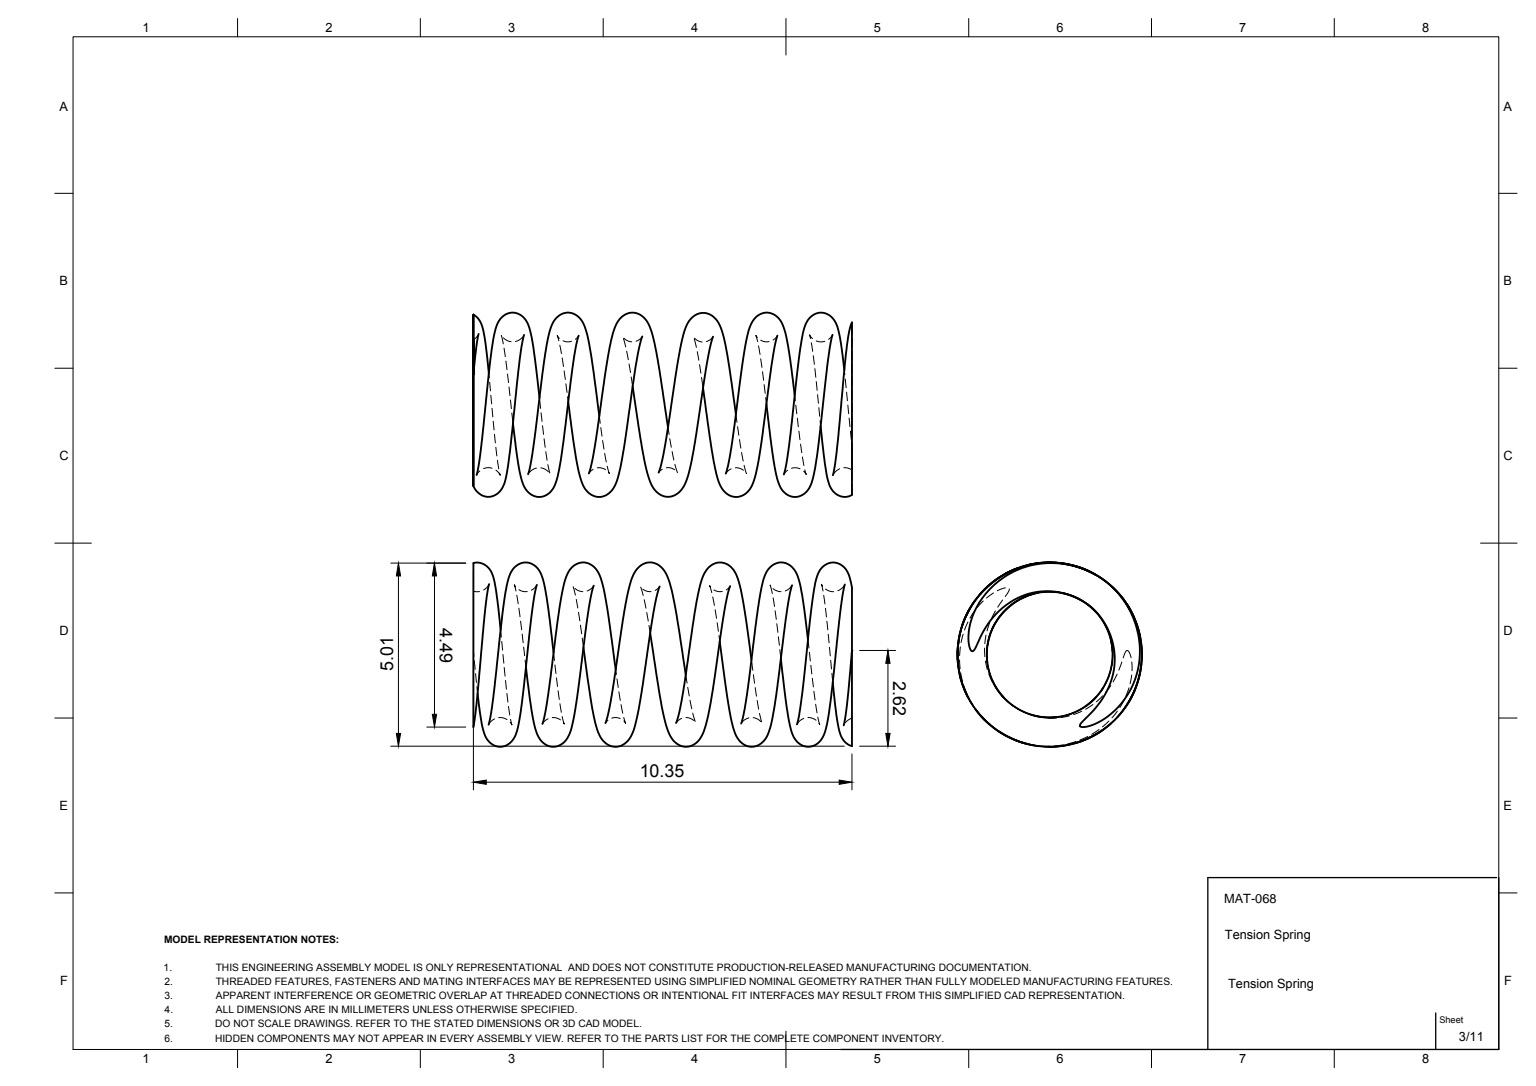
ISO-10303-21;
HEADER;
/* Generated by software containing ST-Developer
 * from STEP Tools, Inc. (www.steptools.com) 
 */

FILE_DESCRIPTION(
/* description */ ('CAx-IF Rec.Pracs.---Representation and Presentation of Product Manufa
cturing Information (PMI)---4.0---2014-10-13'),
/* implementation_level */ '2;1');

FILE_NAME(
/* name */ 'Tension Spring.step',
/* time_stamp */ '2026-10-24T16:53:48-07:00',
/* author */ (''),
/* organization */ (''),
/* preprocessor_version */ 'ST-DEVELOPER v20.2',
/* originating_system */ 'Autodesk Translation Framework v15.17.0.0',
/* authorisation */ '');

FILE_SCHEMA (('AP242_MANAGED_MODEL_BASED_3D_ENGINEERING_MIM_LF { 1 0 10303 442 2 1 4 }'));
ENDSEC;

DATA;
#10=MECHANICAL_DESIGN_GEOMETRIC_PRESENTATION_REPRESENTATION('',(#3490),#107910);
#1137=B_SPLINE_CURVE_WITH_KNOTS('',3,(#63074,#63075,#63076,#63077,#63078,
#63079,#63080,#63081,#63082,#63083,#63084,#63085,#63086,#63087,#63088,#63089,
#63090,#63091,#63092,#63093,#63094,#63095,#63096,#63097,#63098,#63099,#63100,
#63101,#63102,#63103,#63104,#63105,#63106,#63107,#63108,#63109,#63110,#63111,
#63112,#63113,#63114,#63115,#63116,#63117,#63118,#63119,#63120,#63121,#63122,
#63123,#63124,#63125,#63126,#63127,#63128,#63129,#63130,#63131,#63132,#63133,
#63134,#63135,#63136,#63137,#63138,#63139,#63140,#63141,#63142,#63143,#63144,
#63145,#63146,#63147,#63148,#63149,#63150,#63151,#63152,#63153,#63154,#63155,
#63156),.UNSPECIFIED.,.T.,.F.,(4,2,2,2,2,2,2,2,2,2,2,2,3,2,2,2,2,2,2,2,
2,2,2,2,2,2,2,2,2,2,2,2,2,2,2,2,2,2,2,2,4),(-0.599947803193285,-0.598210079042782,
-0.595023554691837,-0.589519553668659,-0.577119648198067,-0.557048780033889,
-0.513453225651634,-0.469622814326577,-0.408953064788174,-0.324588709422408,
-0.21162571525016,-0.096634471246167,0.,0.0616122332173725,0.106433599409592,
0.154580821050161,0.198356973080929,0.2347927451485,0.252280410989761,0.259282926921628,
0.262487356696865,0.264544192713024,0.266469924405381,0.268877657633077,
0.272576047854324,0.281287606126543,0.323717973586198,0.361493711229503,
0.406553787309279,0.452201240933876,0.498262558787684,0.554089254539195,
0.609870344197402,0.658248710788607,0.705297953991042,0.768328967391763,
0.788964957538382,0.796607886518312,0.800333694334371,0.802819259400907,
0.803509190912599),.UNSPECIFIED.);
#1138=B_SPLINE_CURVE_WITH_KNOTS('',3,(#63158,#63159,#63160,#63161,#63162,
#63163,#63164,#63165,#63166,#63167,#63168,#63169,#63170,#63171,#63172,#63173,
#63174,#63175,#63176,#63177,#63178,#63179,#63180,#63181,#63182,#63183,#63184,
#63185,#63186,#63187,#63188,#63189,#63190,#63191,#63192,#63193,#63194,#63195,
#63196,#63197,#63198,#63199,#63200,#63201,#63202,#63203,#63204,#63205,#63206,
#63207,#63208,#63209,#63210,#63211,#63212,#63213,#63214,#63215,#63216,#63217,
#63218,#63219,#63220,#63221,#63222,#63223,#63224,#63225,#63226,#63227,#63228,
#63229,#63230,#63231,#63232,#63233,#63234,#63235,#63236,#63237,#63238,#63239,
#63240,#63241,#63242,#63243,#63244,#63245,#63246,#63247,#63248,#63249,#63250,
#63251,#63252,#63253,#63254,#63255,#63256,#63257,#63258,#63259,#63260,#63261,
#63262,#63263,#63264,#63265,#63266,#63267,#63268,#63269,#63270,#63271,#63272,
#63273),.UNSPECIFIED.,.F.,.F.,(4,2,2,2,2,2,2,2,2,2,2,2,2,2,2,2,2,2,2,2,
2,2,2,2,2,2,2,2,2,2,2,2,2,2,2,2,2,2,2,2,2,2,2,2,2,2,2,2,2,2,2,2,2,2,2,2,
2,4),(-0.961745163027192,-0.959551497797208,-0.949439372246509,-0.939327246695811,
-0.929215121145113,-0.919102995594415,-0.90600602698209,-0.892909058369764,
-0.879812089757439,-0.866715121145113,-0.853618152532788,-0.840521183920462,
-0.827424215308137,-0.814327246695811,-0.801230278083486,-0.78813330947116,
-0.775036340858835,-0.761939372246509,-0.748842403634184,-0.735745435021858,
-0.722648466409533,-0.709551497797208,-0.696454529184882,-0.683357560572557,
-0.670260591960231,-0.657163623347906,-0.630969686123255,-0.604775748898604,
-0.578581811673953,-0.552387874449302,-0.526193937224651,-0.5,-0.484375,
-0.46875,-0.453125,-0.4375,-0.421875,-0.40625,-0.390625,-0.375,-0.359375,
-0.34375,-0.328125,-0.3125,-0.296875,-0.28125,-0.265625,-0.25,-0.234375,
-0.21875,-0.203125,-0.1875,-0.171875,-0.15625,-0.140625,-0.125,-0.109375,
-0.0989179337808057),.UNSPECIFIED.);
#1139=B_SPLINE_CURVE_WITH_KNOTS('',3,(#63275,#63276,#63277,#63278,#63279,
#63280,#63281,#63282,#63283,#63284,#63285,#63286,#63287,#63288,#63289,#63290,
#63291,#63292,#63293,#63294,#63295,#63296,#63297,#63298,#63299,#63300,#63301,
#63302,#63303,#63304,#63305,#63306,#63307,#63308,#63309,#63310,#63311,#63312,
#63313,#63314,#63315,#63316,#63317,#63318,#63319,#63320),.UNSPECIFIED.,
 .F.,.F.,(4,2,2,2,2,2,2,2,2,2,2,2,2,2,2,2,2,2,2,2,2,2,4),(-0.312874562310564,
-0.312343318679824,-0.311777586933697,-0.310438784231193,-0.306394877451961,
-0.293785182499551,-0.270387674138583,-0.246836971206823,-0.225592982310943,
-0.204563523252551,-0.183676969037245,-0.162538995601613,-0.140338814786806,
-0.119352240670363,-0.0971458868601155,-0.0708223711118798,-0.0453771530160624,
-0.0210971413466181,-0.00826159404632588,-0.00338196220690753,-0.00156167910744416,
-0.000763386858963189,-1.00001651581749E-6),.UNSPECIFIED.);
#1140=B_SPLINE_CURVE_WITH_KNOTS('',3,(#63321,#63322,#63323,#63324,#63325,
#63326,#63327,#63328,#63329,#63330,#63331,#63332,#63333,#63334,#63335,#63336,
#63337,#63338,#63339,#63340,#63341,#63342,#63343,#63344,#63345,#63346,#63347,
#63348,#63349,#63350,#63351,#63352,#63353,#63354,#63355,#63356,#63357,#63358,
#63359,#63360,#63361,#63362),.UNSPECIFIED.,.F.,.F.,(4,2,2,2,2,2,2,2,2,2,
2,2,2,2,2,2,2,2,2,2,4),(-0.324422676430501,-0.322867183051822,-0.321207977750209,
-0.317288633341995,-0.30789162270818,-0.28791232922133,-0.250322309326329,
-0.219033304596212,-0.190889649268595,-0.159649528873206,-0.130027804319714,
-0.101827459859418,-0.0752726588112276,-0.0561355587291201,-0.0422771346435577,
-0.0237288423555526,-0.01099220502612,-0.00489383549143937,-0.00219752038096737,
-0.00104712084043852,-1.00002643327324E-6),.UNSPECIFIED.);
#2198=B_SPLINE_SURFACE_WITH_KNOTS('',3,3,((#61813,#61814,#61815,#61816,
#61817,#61818,#61819,#61820,#61821,#61822,#61823,#61824,#61825,#61826,#61827,
#61828,#61829,#61830,#61831,#61832,#61833,#61834,#61835,#61836,#61837,#61838,
#61839,#61840,#61841,#61842,#61843,#61844,#61845,#61846,#61847,#61848,#61849,
#61850,#61851,#61852,#61853,#61854,#61855,#61856,#61857,#61858,#61859,#61860,
#61861,#61862,#61863,#61864,#61865,#61866,#61867,#61868,#61869,#61870,#61871,
#61872,#61873,#61874,#61875,#61876,#61877,#61878,#61879,#61880,#61881,#61882,
#61883,#61884,#61885,#61886,#61887,#61888,#61889,#61890,#61891,#61892,#61893,
#61894,#61895,#61896,#61897,#61898,#61899,#61900,#61901,#61902,#61903,#61904,
#61905,#61906,#61907,#61908,#61909,#61910,#61911,#61912,#61913,#61914,#61915,
#61916,#61917,#61918,#61919,#61920,#61921,#61922,#61923,#61924,#61925,#61926,
#61927,#61928,#61929,#61930,#61931,#61932,#61933,#61934,#61935,#61936,#61937,
#61938),(#61939,#61940,#61941,#61942,#61943,#61944,#61945,#61946,#61947,
#61948,#61949,#61950,#61951,#61952,#61953,#61954,#61955,#61956,#61957,#61958,
#61959,#61960,#61961,#61962,#61963,#61964,#61965,#61966,#61967,#61968,#61969,
#61970,#61971,#61972,#61973,#61974,#61975,#61976,#61977,#61978,#61979,#61980,
#61981,#61982,#61983,#61984,#61985,#61986,#61987,#61988,#61989,#61990,#61991,
#61992,#61993,#61994,#61995,#61996,#61997,#61998,#61999,#62000,#62001,#62002,
#62003,#62004,#62005,#62006,#62007,#62008,#62009,#62010,#62011,#62012,#62013,
#62014,#62015,#62016,#62017,#62018,#62019,#62020,#62021,#62022,#62023,#62024,
#62025,#62026,#62027,#62028,#62029,#62030,#62031,#62032,#62033,#62034,#62035,
#62036,#62037,#62038,#62039,#62040,#62041,#62042,#62043,#62044,#62045,#62046,
#62047,#62048,#62049,#62050,#62051,#62052,#62053,#62054,#62055,#62056,#62057,
#62058,#62059,#62060,#62061,#62062,#62063,#62064),(#62065,#62066,#62067,
#62068,#62069,#62070,#62071,#62072,#62073,#62074,#62075,#62076,#62077,#62078,
#62079,#62080,#62081,#62082,#62083,#62084,#62085,#62086,#62087,#62088,#62089,
#62090,#62091,#62092,#62093,#62094,#62095,#62096,#62097,#62098,#62099,#62100,
#62101,#62102,#62103,#62104,#62105,#62106,#62107,#62108,#62109,#62110,#62111,
#62112,#62113,#62114,#62115,#62116,#62117,#62118,#62119,#62120,#62121,#62122,
#62123,#62124,#62125,#62126,#62127,#62128,#62129,#62130,#62131,#62132,#62133,
#62134,#62135,#62136,#62137,#62138,#62139,#62140,#62141,#62142,#62143,#62144,
#62145,#62146,#62147,#62148,#62149,#62150,#62151,#62152,#62153,#62154,#62155,
#62156,#62157,#62158,#62159,#62160,#62161,#62162,#62163,#62164,#62165,#62166,
#62167,#62168,#62169,#62170,#62171,#62172,#62173,#62174,#62175,#62176,#62177,
#62178,#62179,#62180,#62181,#62182,#62183,#62184,#62185,#62186,#62187,#62188,
#62189,#62190),(#62191,#62192,#62193,#62194,#62195,#62196,#62197,#62198,
#62199,#62200,#62201,#62202,#62203,#62204,#62205,#62206,#62207,#62208,#62209,
#62210,#62211,#62212,#62213,#62214,#62215,#62216,#62217,#62218,#62219,#62220,
#62221,#62222,#62223,#62224,#62225,#62226,#62227,#62228,#62229,#62230,#62231,
#62232,#62233,#62234,#62235,#62236,#62237,#62238,#62239,#62240,#62241,#62242,
#62243,#62244,#62245,#62246,#62247,#62248,#62249,#62250,#62251,#62252,#62253,
#62254,#62255,#62256,#62257,#62258,#62259,#62260,#62261,#62262,#62263,#62264,
#62265,#62266,#62267,#62268,#62269,#62270,#62271,#62272,#62273,#62274,#62275,
#62276,#62277,#62278,#62279,#62280,#62281,#62282,#62283,#62284,#62285,#62286,
#62287,#62288,#62289,#62290,#62291,#62292,#62293,#62294,#62295,#62296,#62297,
#62298,#62299,#62300,#62301,#62302,#62303,#62304,#62305,#62306,#62307,#62308,
#62309,#62310,#62311,#62312,#62313,#62314,#62315,#62316),(#62317,#62318,
#62319,#62320,#62321,#62322,#62323,#62324,#62325,#62326,#62327,#62328,#62329,
#62330,#62331,#62332,#62333,#62334,#62335,#62336,#62337,#62338,#62339,#62340,
#62341,#62342,#62343,#62344,#62345,#62346,#62347,#62348,#62349,#62350,#62351,
#62352,#62353,#62354,#62355,#62356,#62357,#62358,#62359,#62360,#62361,#62362,
#62363,#62364,#62365,#62366,#62367,#62368,#62369,#62370,#62371,#62372,#62373,
#62374,#62375,#62376,#62377,#62378,#62379,#62380,#62381,#62382,#62383,#62384,
#62385,#62386,#62387,#62388,#62389,#62390,#62391,#62392,#62393,#62394,#62395,
#62396,#62397,#62398,#62399,#62400,#62401,#62402,#62403,#62404,#62405,#62406,
#62407,#62408,#62409,#62410,#62411,#62412,#62413,#62414,#62415,#62416,#62417,
#62418,#62419,#62420,#62421,#62422,#62423,#62424,#62425,#62426,#62427,#62428,
#62429,#62430,#62431,#62432,#62433,#62434,#62435,#62436,#62437,#62438,#62439,
#62440,#62441,#62442),(#62443,#62444,#62445,#62446,#62447,#62448,#62449,
#62450,#62451,#62452,#62453,#62454,#62455,#62456,#62457,#62458,#62459,#62460,
#62461,#62462,#62463,#62464,#62465,#62466,#62467,#62468,#62469,#62470,#62471,
#62472,#62473,#62474,#62475,#62476,#62477,#62478,#62479,#62480,#62481,#62482,
#62483,#62484,#62485,#62486,#62487,#62488,#62489,#62490,#62491,#62492,#62493,
#62494,#62495,#62496,#62497,#62498,#62499,#62500,#62501,#62502,#62503,#62504,
#62505,#62506,#62507,#62508,#62509,#62510,#62511,#62512,#62513,#62514,#62515,
#62516,#62517,#62518,#62519,#62520,#62521,#62522,#62523,#62524,#62525,#62526,
#62527,#62528,#62529,#62530,#62531,#62532,#62533,#62534,#62535,#62536,#62537,
#62538,#62539,#62540,#62541,#62542,#62543,#62544,#62545,#62546,#62547,#62548,
#62549,#62550,#62551,#62552,#62553,#62554,#62555,#62556,#62557,#62558,#62559,
#62560,#62561,#62562,#62563,#62564,#62565,#62566,#62567,#62568),(#62569,
#62570,#62571,#62572,#62573,#62574,#62575,#62576,#62577,#62578,#62579,#62580,
#62581,#62582,#62583,#62584,#62585,#62586,#62587,#62588,#62589,#62590,#62591,
#62592,#62593,#62594,#62595,#62596,#62597,#62598,#62599,#62600,#62601,#62602,
#62603,#62604,#62605,#62606,#62607,#62608,#62609,#62610,#62611,#62612,#62613,
#62614,#62615,#62616,#62617,#62618,#62619,#62620,#62621,#62622,#62623,#62624,
#62625,#62626,#62627,#62628,#62629,#62630,#62631,#62632,#62633,#62634,#62635,
#62636,#62637,#62638,#62639,#62640,#62641,#62642,#62643,#62644,#62645,#62646,
#62647,#62648,#62649,#62650,#62651,#62652,#62653,#62654,#62655,#62656,#62657,
#62658,#62659,#62660,#62661,#62662,#62663,#62664,#62665,#62666,#62667,#62668,
#62669,#62670,#62671,#62672,#62673,#62674,#62675,#62676,#62677,#62678,#62679,
#62680,#62681,#62682,#62683,#62684,#62685,#62686,#62687,#62688,#62689,#62690,
#62691,#62692,#62693,#62694),(#62695,#62696,#62697,#62698,#62699,#62700,
#62701,#62702,#62703,#62704,#62705,#62706,#62707,#62708,#62709,#62710,#62711,
#62712,#62713,#62714,#62715,#62716,#62717,#62718,#62719,#62720,#62721,#62722,
#62723,#62724,#62725,#62726,#62727,#62728,#62729,#62730,#62731,#62732,#62733,
#62734,#62735,#62736,#62737,#62738,#62739,#62740,#62741,#62742,#62743,#62744,
#62745,#62746,#62747,#62748,#62749,#62750,#62751,#62752,#62753,#62754,#62755,
#62756,#62757,#62758,#62759,#62760,#62761,#62762,#62763,#62764,#62765,#62766,
#62767,#62768,#62769,#62770,#62771,#62772,#62773,#62774,#62775,#62776,#62777,
#62778,#62779,#62780,#62781,#62782,#62783,#62784,#62785,#62786,#62787,#62788,
#62789,#62790,#62791,#62792,#62793,#62794,#62795,#62796,#62797,#62798,#62799,
#62800,#62801,#62802,#62803,#62804,#62805,#62806,#62807,#62808,#62809,#62810,
#62811,#62812,#62813,#62814,#62815,#62816,#62817,#62818,#62819,#62820),
(#62821,#62822,#62823,#62824,#62825,#62826,#62827,#62828,#62829,#62830,
#62831,#62832,#62833,#62834,#62835,#62836,#62837,#62838,#62839,#62840,#62841,
#62842,#62843,#62844,#62845,#62846,#62847,#62848,#62849,#62850,#62851,#62852,
#62853,#62854,#62855,#62856,#62857,#62858,#62859,#62860,#62861,#62862,#62863,
#62864,#62865,#62866,#62867,#62868,#62869,#62870,#62871,#62872,#62873,#62874,
#62875,#62876,#62877,#62878,#62879,#62880,#62881,#62882,#62883,#62884,#62885,
#62886,#62887,#62888,#62889,#62890,#62891,#62892,#62893,#62894,#62895,#62896,
#62897,#62898,#62899,#62900,#62901,#62902,#62903,#62904,#62905,#62906,#62907,
#62908,#62909,#62910,#62911,#62912,#62913,#62914,#62915,#62916,#62917,#62918,
#62919,#62920,#62921,#62922,#62923,#62924,#62925,#62926,#62927,#62928,#62929,
#62930,#62931,#62932,#62933,#62934,#62935,#62936,#62937,#62938,#62939,#62940,
#62941,#62942,#62943,#62944,#62945,#62946),(#62947,#62948,#62949,#62950,
#62951,#62952,#62953,#62954,#62955,#62956,#62957,#62958,#62959,#62960,#62961,
#62962,#62963,#62964,#62965,#62966,#62967,#62968,#62969,#62970,#62971,#62972,
#62973,#62974,#62975,#62976,#62977,#62978,#62979,#62980,#62981,#62982,#62983,
#62984,#62985,#62986,#62987,#62988,#62989,#62990,#62991,#62992,#62993,#62994,
#62995,#62996,#62997,#62998,#62999,#63000,#63001,#63002,#63003,#63004,#63005,
#63006,#63007,#63008,#63009,#63010,#63011,#63012,#63013,#63014,#63015,#63016,
#63017,#63018,#63019,#63020,#63021,#63022,#63023,#63024,#63025,#63026,#63027,
#63028,#63029,#63030,#63031,#63032,#63033,#63034,#63035,#63036,#63037,#63038,
#63039,#63040,#63041,#63042,#63043,#63044,#63045,#63046,#63047,#63048,#63049,
#63050,#63051,#63052,#63053,#63054,#63055,#63056,#63057,#63058,#63059,#63060,
#63061,#63062,#63063,#63064,#63065,#63066,#63067,#63068,#63069,#63070,#63071,
#63072)),.UNSPECIFIED.,.T.,.F.,.F.,(4,2,2,2,4),(4,2,2,2,2,2,2,2,2,2,2,2,
2,2,2,2,2,2,2,2,2,2,2,2,2,2,2,2,2,2,2,2,2,2,2,2,2,2,2,2,2,2,2,2,2,2,2,2,
2,2,2,2,2,2,2,2,2,2,2,2,2,2,4),(0.,0.25,0.5,0.75,1.),(0.0266743037386738,
0.03125,0.046875,0.0625,0.078125,0.09375,0.109375,0.125,0.140625,0.15625,
0.171875,0.1875,0.203125,0.21875,0.234375,0.25,0.265625,0.28125,0.296875,
0.3125,0.328125,0.34375,0.359375,0.375,0.390625,0.40625,0.421875,0.4375,
0.453125,0.46875,0.484375,0.5,0.526193937224651,0.552387874449302,0.578581811673953,
0.604775748898604,0.630969686123255,0.657163623347906,0.670260591960231,
0.683357560572557,0.696454529184882,0.709551497797208,0.722648466409533,
0.735745435021858,0.748842403634184,0.761939372246509,0.775036340858835,
0.78813330947116,0.801230278083486,0.814327246695811,0.827424215308137,
0.840521183920462,0.853618152532788,0.866715121145113,0.879812089757439,
0.892909058369764,0.90600602698209,0.919102995594415,0.929215121145113,
0.939327246695811,0.949439372246509,0.959551497797208,0.967322126402602),
 .UNSPECIFIED.);
#3470=SHAPE_REPRESENTATION_RELATIONSHIP('SRR','None',#107948,#3480);
#3480=ADVANCED_BREP_SHAPE_REPRESENTATION('',(#3500),#107901);
#3490=STYLED_ITEM('',(#108007),#3500);
#3500=MANIFOLD_SOLID_BREP('Body1',#45538);
#3544=PLANE('',#45669);
#3545=PLANE('',#45670);
#3762=FACE_OUTER_BOUND('',#6688,.T.);
#3763=FACE_OUTER_BOUND('',#6689,.T.);
#3764=FACE_OUTER_BOUND('',#6690,.T.);
#6688=EDGE_LOOP('',(#28134,#28135,#28136,#28137,#28138));
#6689=EDGE_LOOP('',(#28139,#28140));
#6690=EDGE_LOOP('',(#28141));
#17183=VERTEX_POINT('',#63073);
#17184=VERTEX_POINT('',#63157);
#17185=VERTEX_POINT('',#63274);
#21209=EDGE_CURVE('',#17183,#17183,#1137,.F.);
#21210=EDGE_CURVE('',#17183,#17184,#1138,.T.);
#21211=EDGE_CURVE('',#17184,#17185,#1139,.F.);
#21212=EDGE_CURVE('',#17185,#17184,#1140,.F.);
#28134=ORIENTED_EDGE('',*,*,#21209,.T.);
#28135=ORIENTED_EDGE('',*,*,#21210,.T.);
#28136=ORIENTED_EDGE('',*,*,#21211,.T.);
#28137=ORIENTED_EDGE('',*,*,#21212,.T.);
#28138=ORIENTED_EDGE('',*,*,#21210,.F.);
#28139=ORIENTED_EDGE('',*,*,#21211,.F.);
#28140=ORIENTED_EDGE('',*,*,#21212,.F.);
#28141=ORIENTED_EDGE('',*,*,#21209,.F.);
#42617=ADVANCED_FACE('',(#3762),#2198,.T.);
#42618=ADVANCED_FACE('',(#3763),#3544,.T.);
#42619=ADVANCED_FACE('',(#3764),#3545,.T.);
#45538=CLOSED_SHELL('',(#42617,#42618,#42619));
#45668=AXIS2_PLACEMENT_3D('',#61812,#50398,#50399);
#45669=AXIS2_PLACEMENT_3D('',#63363,#50400,#50401);
#45670=AXIS2_PLACEMENT_3D('',#63364,#50402,#50403);
#50398=DIRECTION('axis',(0.,0.,1.));
#50399=DIRECTION('refdir',(1.,0.,0.));
#50400=DIRECTION('center_axis',(-3.37541892033393E-34,1.,-4.11561597259898E-17));
#50401=DIRECTION('ref_axis',(1.,-1.28292706084425E-49,-8.20149144819841E-18));
#50402=DIRECTION('center_axis',(-1.19904736293711E-16,-1.,2.51898569257898E-21));
#50403=DIRECTION('ref_axis',(-1.,1.19904736293711E-16,0.));
#61812=CARTESIAN_POINT('',(0.,0.,0.));
#61813=CARTESIAN_POINT('Ctrl Pts',(0.00815067148752137,-0.0203072579114564,
0.0762656663521488));
#61814=CARTESIAN_POINT('Ctrl Pts',(0.0083771381325318,-0.0203255606965017,
0.0762649347079084));
#61815=CARTESIAN_POINT('Ctrl Pts',(0.00860198035030984,-0.0203438634815471,
0.0762288078613937));
#61816=CARTESIAN_POINT('Ctrl Pts',(0.00953656982276594,-0.0204246662665928,
0.0759073888491967));
#61817=CARTESIAN_POINT('Ctrl Pts',(0.0100801851138304,-0.0204871662665918,
0.0752518676024789));
#61818=CARTESIAN_POINT('Ctrl Pts',(0.0103422385382883,-0.0206121662665931,
0.0738034800723812));
#61819=CARTESIAN_POINT('Ctrl Pts',(0.0100648920002843,-0.020674666266593,
0.0730378901277388));
#61820=CARTESIAN_POINT('Ctrl Pts',(0.00900362893656076,-0.0207996662665919,
0.0720931661776728));
#61821=CARTESIAN_POINT('Ctrl Pts',(0.008241028020177,-0.0208621662665925,
0.0719231783970233));
#61822=CARTESIAN_POINT('Ctrl Pts',(0.00691275415584957,-0.0209871662665924,
0.0722775972279668));
#61823=CARTESIAN_POINT('Ctrl Pts',(0.00636364311727103,-0.0210496662665924,
0.0727913084945308));
#61824=CARTESIAN_POINT('Ctrl Pts',(0.00590286642913209,-0.0211746662665925,
0.0740419937307385));
#61825=CARTESIAN_POINT('Ctrl Pts',(0.00599202908596152,-0.0212371662665924,
0.0747620631556615));
#61826=CARTESIAN_POINT('Ctrl Pts',(0.00669689975963152,-0.0213621662665925,
0.0758479396774564));
#61827=CARTESIAN_POINT('Ctrl Pts',(0.00730138706368173,-0.0214246662665922,
0.0762043156608544));
#61828=CARTESIAN_POINT('Ctrl Pts',(0.00855547426588603,-0.0215496662665927,
0.0763202968801402));
#61829=CARTESIAN_POINT('Ctrl Pts',(0.00919252612250013,-0.0216121662665926,
0.0760823999614819));
#61830=CARTESIAN_POINT('Ctrl Pts',(0.0100589999732895,-0.0217371662665924,
0.075213633090309));
#61831=CARTESIAN_POINT('Ctrl Pts',(0.0102830084237745,-0.0217996662665926,
0.0745926208223076));
#61832=CARTESIAN_POINT('Ctrl Pts',(0.0101959629269755,-0.0219246662665924,
0.0733988421450626));
#61833=CARTESIAN_POINT('Ctrl Pts',(0.00988830420246689,-0.0219871662665922,
0.0728354269849725));
#61834=CARTESIAN_POINT('Ctrl Pts',(0.00896597799697031,-0.0221121662665928,
0.0721171826520367));
#61835=CARTESIAN_POINT('Ctrl Pts',(0.00835948988205837,-0.022174666266592,
0.0719657358996911));
#61836=CARTESIAN_POINT('Ctrl Pts',(0.00723038395375605,-0.0222996662665929,
0.0721429107222321));
#61837=CARTESIAN_POINT('Ctrl Pts',(0.00671499560243656,-0.0223621662665927,
0.0724683075554325));
#61838=CARTESIAN_POINT('Ctrl Pts',(0.00606901592181546,-0.0224871662665922,
0.0733814268319492));
#61839=CARTESIAN_POINT('Ctrl Pts',(0.00594091088577522,-0.0225496662665926,
0.0739624842354635));
#61840=CARTESIAN_POINT('Ctrl Pts',(0.00612305344798784,-0.0226746662665923,
0.0750428459007938));
#61841=CARTESIAN_POINT('Ctrl Pts',(0.00643067872875265,-0.0227371662665921,
0.0755362893544149));
#61842=CARTESIAN_POINT('Ctrl Pts',(0.00729424742007936,-0.0228621662665928,
0.0761749122408133));
#61843=CARTESIAN_POINT('Ctrl Pts',(0.00784480408877878,-0.0229246662665925,
0.0763178915621161));
#61844=CARTESIAN_POINT('Ctrl Pts',(0.00889151097164585,-0.0230496662665924,
0.0761965031486893));
#61845=CARTESIAN_POINT('Ctrl Pts',(0.00938270763587042,-0.0231121662665924,
0.0759340000649118));
#61846=CARTESIAN_POINT('Ctrl Pts',(0.0100625879641978,-0.0232371662665925,
0.0751542816790953));
#61847=CARTESIAN_POINT('Ctrl Pts',(0.0102490546008787,-0.0232996662665926,
0.0746413589041057));
#61848=CARTESIAN_POINT('Ctrl Pts',(0.0102410178141923,-0.0234246662665924,
0.0736250907589115));
#61849=CARTESIAN_POINT('Ctrl Pts',(0.0100475843126518,-0.0234871662665927,
0.0731260381541277));
#61850=CARTESIAN_POINT('Ctrl Pts',(0.00938855725198137,-0.0236121662665922,
0.0723752164881653));
#61851=CARTESIAN_POINT('Ctrl Pts',(0.0089262758271642,-0.0236746662665927,
0.0721258013564626));
#61852=CARTESIAN_POINT('Ctrl Pts',(0.00795468689116961,-0.0237996662665922,
0.0719791054916663));
#61853=CARTESIAN_POINT('Ctrl Pts',(0.00744911026789867,-0.0238621662665923,
0.0720815291713897));
#61854=CARTESIAN_POINT('Ctrl Pts',(0.00661942895548025,-0.0239871662665926,
0.0725781618664859));
#61855=CARTESIAN_POINT('Ctrl Pts',(0.00629781787585632,-0.0240496662665925,
0.0729699778138594));
#61856=CARTESIAN_POINT('Ctrl Pts',(0.00596869167054677,-0.0241746662665925,
0.07386332441141));
#61857=CARTESIAN_POINT('Ctrl Pts',(0.00596159400885685,-0.0242371662665925,
0.0743616829432692));
#61858=CARTESIAN_POINT('Ctrl Pts',(0.00625226027464946,-0.0243621662665925,
0.0752533010137793));
#61859=CARTESIAN_POINT('Ctrl Pts',(0.0065485129249735,-0.0244246662665925,
0.0756440052932471));
#61860=CARTESIAN_POINT('Ctrl Pts',(0.00731262787164867,-0.0245496662665925,
0.0761638405487234));
#61861=CARTESIAN_POINT('Ctrl Pts',(0.00777792798085125,-0.0246121662665926,
0.0762919438047406));
#61862=CARTESIAN_POINT('Ctrl Pts',(0.00868784969457759,-0.0247371662665924,
0.07624508144423));
#61863=CARTESIAN_POINT('Ctrl Pts',(0.00912998835433636,-0.024799666266592,
0.0760707882292855));
#61864=CARTESIAN_POINT('Ctrl Pts',(0.00982231809848441,-0.024924666266593,
0.07549790728317));
#61865=CARTESIAN_POINT('Ctrl Pts',(0.010071019077723,-0.0249871662665926,
0.0751012030151419));
#61866=CARTESIAN_POINT('Ctrl Pts',(0.0102889821151069,-0.0251121662665924,
0.0742418039415068));
#61867=CARTESIAN_POINT('Ctrl Pts',(0.0102581523851926,-0.0251746662665924,
0.0737813536046464));
#61868=CARTESIAN_POINT('Ctrl Pts',(0.00993809892066803,-0.0252996662665926,
0.0729669145852015));
#61869=CARTESIAN_POINT('Ctrl Pts',(0.00965002750714532,-0.0253621662665928,
0.0726146871985494));
#61870=CARTESIAN_POINT('Ctrl Pts',(0.00892808254078336,-0.0254871662665921,
0.07214009674052));
#61871=CARTESIAN_POINT('Ctrl Pts',(0.00849604407482765,-0.0255496662665926,
0.0720184647612599));
#61872=CARTESIAN_POINT('Ctrl Pts',(0.00764304374228332,-0.0256746662665924,
0.0720402815521564));
#61873=CARTESIAN_POINT('Ctrl Pts',(0.00722389165927775,-0.0257371662665915,
0.0721833149981475));
#61874=CARTESIAN_POINT('Ctrl Pts',(0.00654039915241529,-0.0258621662665935,
0.0726767209970879));
#61875=CARTESIAN_POINT('Ctrl Pts',(0.00627724799864211,-0.0259246662665926,
0.0730258105884879));
#61876=CARTESIAN_POINT('Ctrl Pts',(0.00589186280469173,-0.0260919420154909,
0.0740718608505132));
#61877=CARTESIAN_POINT('Ctrl Pts',(0.00599991759097347,-0.0261967177643892,
0.0748547737082654));
#61878=CARTESIAN_POINT('Ctrl Pts',(0.00685580966361203,-0.0264062692621874,
0.0759938417732247));
#61879=CARTESIAN_POINT('Ctrl Pts',(0.00759343482402584,-0.0265110450110865,
0.0763289629385248));
#61880=CARTESIAN_POINT('Ctrl Pts',(0.00904218730885863,-0.0267205965088817,
0.0761958934123178));
#61881=CARTESIAN_POINT('Ctrl Pts',(0.00972755157183108,-0.0268253722577806,
0.0757250048942655));
#61882=CARTESIAN_POINT('Ctrl Pts',(0.010359884849577,-0.0270349237555792,
0.0743792630330001));
#61883=CARTESIAN_POINT('Ctrl Pts',(0.0102896623256786,-0.0271396995044774,
0.0735275482799331));
#61884=CARTESIAN_POINT('Ctrl Pts',(0.00940073146439328,-0.0273492510022741,
0.0722931522835415));
#61885=CARTESIAN_POINT('Ctrl Pts',(0.00859517611493118,-0.0274540267511745,
0.0719398966766563));
#61886=CARTESIAN_POINT('Ctrl Pts',(0.00705289958900958,-0.0276635782489686,
0.0721600303097132));
#61887=CARTESIAN_POINT('Ctrl Pts',(0.00635232687879448,-0.0277683539978693,
0.0727358184526565));
#61888=CARTESIAN_POINT('Ctrl Pts',(0.00598272505460037,-0.0279255176212164,
0.073875472823177));
#61889=CARTESIAN_POINT('Ctrl Pts',(0.00596897958949985,-0.0279779054956661,
0.0742932638294421));
#61890=CARTESIAN_POINT('Ctrl Pts',(0.00617298034709087,-0.0280826812445643,
0.0750763211850444));
#61891=CARTESIAN_POINT('Ctrl Pts',(0.00639068647810172,-0.0281350691190143,
0.075440160464901));
#61892=CARTESIAN_POINT('Ctrl Pts',(0.00699633121784709,-0.028239844867912,
0.0759930922591544));
#61893=CARTESIAN_POINT('Ctrl Pts',(0.00738340683150901,-0.0282922327423619,
0.0761809264433306));
#61894=CARTESIAN_POINT('Ctrl Pts',(0.00820473003409823,-0.0283970084912602,
0.076310154007468));
#61895=CARTESIAN_POINT('Ctrl Pts',(0.00863746583537968,-0.0284493963657099,
0.0762509280036797));
#61896=CARTESIAN_POINT('Ctrl Pts',(0.00940183247449225,-0.0285541721146081,
0.0758948085378461));
#61897=CARTESIAN_POINT('Ctrl Pts',(0.00973174559026465,-0.028606559989058,
0.0755982633195131));
#61898=CARTESIAN_POINT('Ctrl Pts',(0.0101673721494254,-0.0287113357379557,
0.0748618658679991));
#61899=CARTESIAN_POINT('Ctrl Pts',(0.0102717693088642,-0.0287637236124047,
0.0744233616342778));
#61900=CARTESIAN_POINT('Ctrl Pts',(0.0102064021029961,-0.0288684993613048,
0.0735573200377487));
#61901=CARTESIAN_POINT('Ctrl Pts',(0.0100362994783456,-0.0289208872357529,
0.0731317839731108));
#61902=CARTESIAN_POINT('Ctrl Pts',(0.00947201428442268,-0.0290256629846524,
0.072453899629834));
#61903=CARTESIAN_POINT('Ctrl Pts',(0.00907878062310723,-0.0290780508591023,
0.0722035268267701));
#61904=CARTESIAN_POINT('Ctrl Pts',(0.00821001945932422,-0.0291828266079989,
0.0719835875408627));
#61905=CARTESIAN_POINT('Ctrl Pts',(0.00773657577545569,-0.0292352144824501,
0.0720151544508798));
#61906=CARTESIAN_POINT('Ctrl Pts',(0.00689428236856863,-0.0293399902313469,
0.0723623130857159));
#61907=CARTESIAN_POINT('Ctrl Pts',(0.00652798278812114,-0.029392378105796,
0.0726775538261953));
#61908=CARTESIAN_POINT('Ctrl Pts',(0.00605938394721744,-0.0294971538546968,
0.0734769967671513));
#61909=CARTESIAN_POINT('Ctrl Pts',(0.00595907161542407,-0.0295495417291453,
0.0739592244029917));
#61910=CARTESIAN_POINT('Ctrl Pts',(0.00608211280228693,-0.0296543174780434,
0.0748942803942386));
#61911=CARTESIAN_POINT('Ctrl Pts',(0.00630586837465766,-0.0297067053524937,
0.0753440780020337));
#61912=CARTESIAN_POINT('Ctrl Pts',(0.00699741885923872,-0.0298114811013907,
0.0760106285387534));
#61913=CARTESIAN_POINT('Ctrl Pts',(0.00746350290246076,-0.02986386897584,
0.0762245043065757));
#61914=CARTESIAN_POINT('Ctrl Pts',(0.00843911221849071,-0.0299686447247403,
0.0763040900230327));
#61915=CARTESIAN_POINT('Ctrl Pts',(0.0089451874363639,-0.0300210325991884,
0.0761685265237053));
#61916=CARTESIAN_POINT('Ctrl Pts',(0.00975909850238958,-0.0301258083480876,
0.0755904500898765));
#61917=CARTESIAN_POINT('Ctrl Pts',(0.0100631115942824,-0.0301781962225362,
0.0751492903863319));
#61918=CARTESIAN_POINT('Ctrl Pts',(0.0103054074683059,-0.0302829719714357,
0.0741595369305542));
#61919=CARTESIAN_POINT('Ctrl Pts',(0.0102414483775728,-0.0303353598458849,
0.0736148328055268));
#61920=CARTESIAN_POINT('Ctrl Pts',(0.00975323921825422,-0.0304401355947827,
0.0726954265952984));
#61921=CARTESIAN_POINT('Ctrl Pts',(0.00932997882757754,-0.0304925234692313,
0.0723256171343211));
#61922=CARTESIAN_POINT('Ctrl Pts',(0.00832584380498464,-0.0305972992181321,
0.0719722823282605));
#61923=CARTESIAN_POINT('Ctrl Pts',(0.0077494649754808,-0.0306496870925817,
0.0719920559628832));
#61924=CARTESIAN_POINT('Ctrl Pts',(0.00675592000443203,-0.0307544628414776,
0.0724395062495526));
#61925=CARTESIAN_POINT('Ctrl Pts',(0.00634496891942769,-0.0308068507159279,
0.0728664214919276));
#61926=CARTESIAN_POINT('Ctrl Pts',(0.00594354974162806,-0.0309116264648272,
0.0739084696771727));
#61927=CARTESIAN_POINT('Ctrl Pts',(0.00595750536674637,-0.030964014339277,
0.0745180867156372));
#61928=CARTESIAN_POINT('Ctrl Pts',(0.00638267793035737,-0.0310568507159276,
0.0754400513829074));
#61929=CARTESIAN_POINT('Ctrl Pts',(0.00669956413626623,-0.0310972992181319,
0.0757857300068678));
#61930=CARTESIAN_POINT('Ctrl Pts',(0.00748945302262128,-0.0311781962225358,
0.0762240386264647));
#61931=CARTESIAN_POINT('Ctrl Pts',(0.00796079155782699,-0.0312186447247393,
0.0763148367595518));
#61932=CARTESIAN_POINT('Ctrl Pts',(0.00887509295304323,-0.0312995417291452,
0.0761868152287656));
#61933=CARTESIAN_POINT('Ctrl Pts',(0.00931534986442847,-0.031339990231348,
0.075967462485304));
#61934=CARTESIAN_POINT('Ctrl Pts',(0.00997379973563606,-0.0314208872357532,
0.0752903676969252));
#61935=CARTESIAN_POINT('Ctrl Pts',(0.0101892230058022,-0.0314613357379553,
0.0748339923228011));
#61936=CARTESIAN_POINT('Ctrl Pts',(0.0102708978512695,-0.0315328667545812,
0.0739826395793677));
#61937=CARTESIAN_POINT('Ctrl Pts',(0.0102055680523813,-0.0315639492690025,
0.0735997686615574));
#61938=CARTESIAN_POINT('Ctrl Pts',(0.0100469390803206,-0.0315950317834238,
0.0732561803273014));
#61939=CARTESIAN_POINT('Ctrl Pts',(0.00815332628724061,-0.0203072579114564,
0.0764745476396777));
#61940=CARTESIAN_POINT('Ctrl Pts',(0.00840215214987724,-0.0203255606965017,
0.0764737437596658));
#61941=CARTESIAN_POINT('Ctrl Pts',(0.00864919320439181,-0.0203438634815471,
0.0764340500831514));
#61942=CARTESIAN_POINT('Ctrl Pts',(0.00967605537954476,-0.0204246662665928,
0.0760808971366146));
#61943=CARTESIAN_POINT('Ctrl Pts',(0.0102733422062002,-0.0204871662665918,
0.0753606557973937));
#61944=CARTESIAN_POINT('Ctrl Pts',(0.0105612683570671,-0.0206121662665931,
0.0737692679062889));
#61945=CARTESIAN_POINT('Ctrl Pts',(0.0102565391923597,-0.020674666266593,
0.0729280907060315));
#61946=CARTESIAN_POINT('Ctrl Pts',(0.00909049684955361,-0.0207996662665919,
0.0718900934688763));
#61947=CARTESIAN_POINT('Ctrl Pts',(0.00825260378650262,-0.0208621662665925,
0.0717033226702191));
#61948=CARTESIAN_POINT('Ctrl Pts',(0.00679318847130807,-0.0209871662665924,
0.0720927335317618));
#61949=CARTESIAN_POINT('Ctrl Pts',(0.00618986329796383,-0.0210496662665924,
0.0726571638876892));
#61950=CARTESIAN_POINT('Ctrl Pts',(0.00568359379013531,-0.0211746662665925,
0.0740313301927182));
#61951=CARTESIAN_POINT('Ctrl Pts',(0.00578155954133694,-0.0212371662665924,
0.0748224925990252));
#61952=CARTESIAN_POINT('Ctrl Pts',(0.00655602261255478,-0.0213621662665925,
0.076015578504634));
#61953=CARTESIAN_POINT('Ctrl Pts',(0.00722019139059382,-0.0214246662665922,
0.0764071397497255));
#61954=CARTESIAN_POINT('Ctrl Pts',(0.00859809554021233,-0.0215496662665927,
0.0765345718796849));
#61955=CARTESIAN_POINT('Ctrl Pts',(0.00929804399292574,-0.0216121662665926,
0.0762731872241167));
#61956=CARTESIAN_POINT('Ctrl Pts',(0.010250065441227,-0.0217371662665924,
0.0753186463638511));
#61957=CARTESIAN_POINT('Ctrl Pts',(0.0104961904099933,-0.0217996662665926,
0.0746363211000744));
#61958=CARTESIAN_POINT('Ctrl Pts',(0.0104005508475817,-0.0219246662665924,
0.0733246797802278));
#61959=CARTESIAN_POINT('Ctrl Pts',(0.0100625167520088,-0.0219871662665922,
0.0727056382289851));
#61960=CARTESIAN_POINT('Ctrl Pts',(0.00904912860513842,-0.0221121662665928,
0.0719164811073332));
#61961=CARTESIAN_POINT('Ctrl Pts',(0.00838276147471677,-0.022174666266592,
0.0717500819062757));
#61962=CARTESIAN_POINT('Ctrl Pts',(0.00714217809165384,-0.0222996662665929,
0.0719447493287309));
#61963=CARTESIAN_POINT('Ctrl Pts',(0.0065759050711654,-0.0223621662665927,
0.0723022728294504));
#61964=CARTESIAN_POINT('Ctrl Pts',(0.00586614734384593,-0.0224871662665922,
0.0733055450405034));
#61965=CARTESIAN_POINT('Ctrl Pts',(0.00572539440382979,-0.0225496662665926,
0.073943970666777));
#61966=CARTESIAN_POINT('Ctrl Pts',(0.00592552003453053,-0.0226746662665923,
0.0751309972301058));
#61967=CARTESIAN_POINT('Ctrl Pts',(0.00626351738443437,-0.0227371662665921,
0.0756731587170833));
#61968=CARTESIAN_POINT('Ctrl Pts',(0.00721234684475271,-0.0228621662665928,
0.0763748333085017));
#61969=CARTESIAN_POINT('Ctrl Pts',(0.00781726037633776,-0.0229246662665925,
0.0765319290828517));
#61970=CARTESIAN_POINT('Ctrl Pts',(0.00896730939589689,-0.0230496662665924,
0.076398555902516));
#61971=CARTESIAN_POINT('Ctrl Pts',(0.00950700226631619,-0.0231121662665924,
0.0761101356971356));
#61972=CARTESIAN_POINT('Ctrl Pts',(0.010254007677104,-0.0232371662665925,
0.0752534351443655));
#61973=CARTESIAN_POINT('Ctrl Pts',(0.0104588843013103,-0.0232996662665926,
0.0746898711283627));
#61974=CARTESIAN_POINT('Ctrl Pts',(0.0104500540367917,-0.0234246662665924,
0.0735732660853268));
#61975=CARTESIAN_POINT('Ctrl Pts',(0.0102375227040588,-0.0234871662665927,
0.0730249416515866));
#61976=CARTESIAN_POINT('Ctrl Pts',(0.00951342941930744,-0.0236121662665922,
0.0721999908129729));
#61977=CARTESIAN_POINT('Ctrl Pts',(0.00900550661104702,-0.0236746662665927,
0.0719259507427556));
#61978=CARTESIAN_POINT('Ctrl Pts',(0.00793799198823834,-0.0237996662665922,
0.0717647714878526));
#61979=CARTESIAN_POINT('Ctrl Pts',(0.0073824994148905,-0.0238621662665923,
0.071877307532445));
#61980=CARTESIAN_POINT('Ctrl Pts',(0.00647090305920422,-0.0239871662665926,
0.0724229731370429));
#61981=CARTESIAN_POINT('Ctrl Pts',(0.0061175390822829,-0.0240496662665925,
0.0728534733596938));
#61982=CARTESIAN_POINT('Ctrl Pts',(0.0057559180058162,-0.0241746662665925,
0.0738350207207137));
#61983=CARTESIAN_POINT('Ctrl Pts',(0.00574811958679247,-0.0242371662665925,
0.0743825825552014));
#61984=CARTESIAN_POINT('Ctrl Pts',(0.00606748354576255,-0.0243621662665925,
0.075362230730441));
#61985=CARTESIAN_POINT('Ctrl Pts',(0.00639298543709791,-0.0244246662665925,
0.0757915095294001));
#61986=CARTESIAN_POINT('Ctrl Pts',(0.00723254201175921,-0.0245496662665925,
0.0763626685001477));
#61987=CARTESIAN_POINT('Ctrl Pts',(0.00774378154132399,-0.0246121662665926,
0.0765034194843978));
#61988=CARTESIAN_POINT('Ctrl Pts',(0.00874354049187196,-0.0247371662665924,
0.0764519303687327));
#61989=CARTESIAN_POINT('Ctrl Pts',(0.00922933182513614,-0.024799666266592,
0.0762604290571012));
#61990=CARTESIAN_POINT('Ctrl Pts',(0.00999001579168093,-0.024924666266593,
0.0756309871558503));
#61991=CARTESIAN_POINT('Ctrl Pts',(0.0102632712006387,-0.0249871662665926,
0.0751951159850686));
#61992=CARTESIAN_POINT('Ctrl Pts',(0.0105027538882435,-0.0251121662665924,
0.0742508678118485));
#61993=CARTESIAN_POINT('Ctrl Pts',(0.0104688803165286,-0.0251746662665924,
0.0737449568761991));
#61994=CARTESIAN_POINT('Ctrl Pts',(0.0101172277391856,-0.0252996662665926,
0.0728501076962283));
#61995=CARTESIAN_POINT('Ctrl Pts',(0.00980071482414927,-0.0253621662665928,
0.0724631046418761));
#61996=CARTESIAN_POINT('Ctrl Pts',(0.00900749170282425,-0.0254871662665921,
0.0719416575205446));
#61997=CARTESIAN_POINT('Ctrl Pts',(0.00853279776289023,-0.0255496662665926,
0.0718080167269426));
#61998=CARTESIAN_POINT('Ctrl Pts',(0.0075955800831525,-0.0256746662665924,
0.0718319875055733));
#61999=CARTESIAN_POINT('Ctrl Pts',(0.0071350448081896,-0.0257371662665915,
0.0719891427483816));
#62000=CARTESIAN_POINT('Ctrl Pts',(0.0063840705858361,-0.0258621662665935,
0.0725312630827505));
#62001=CARTESIAN_POINT('Ctrl Pts',(0.00609493832603504,-0.0259246662665926,
0.0729148185450287));
#62002=CARTESIAN_POINT('Ctrl Pts',(0.00567150376979967,-0.0260919420154909,
0.0740641461150897));
#62003=CARTESIAN_POINT('Ctrl Pts',(0.00579022688422278,-0.0261967177643892,
0.0749243565323479));
#62004=CARTESIAN_POINT('Ctrl Pts',(0.00673062180767083,-0.0264062692621874,
0.0761758856211119));
#62005=CARTESIAN_POINT('Ctrl Pts',(0.00754107324008372,-0.0265110450110865,
0.076544093544357));
#62006=CARTESIAN_POINT('Ctrl Pts',(0.00913286211817163,-0.0267205965088817,
0.0763978859664261));
#62007=CARTESIAN_POINT('Ctrl Pts',(0.00988589289648584,-0.0268253722577806,
0.0758805062803154));
#62008=CARTESIAN_POINT('Ctrl Pts',(0.0105806569015859,-0.0270349237555792,
0.0744018983400594));
#62009=CARTESIAN_POINT('Ctrl Pts',(0.0105035012565028,-0.0271396995044774,
0.0734660931660017));
#62010=CARTESIAN_POINT('Ctrl Pts',(0.00952680560062186,-0.0273492510022741,
0.072109824349359));
#62011=CARTESIAN_POINT('Ctrl Pts',(0.00864171718187381,-0.0274540267511745,
0.0717216915578374));
#62012=CARTESIAN_POINT('Ctrl Pts',(0.00694717056566465,-0.0276635782489686,
0.0719635591456149));
#62013=CARTESIAN_POINT('Ctrl Pts',(0.0061774297989796,-0.0277683539978693,
0.0725961952733644));
#62014=CARTESIAN_POINT('Ctrl Pts',(0.00577133691614923,-0.0279255176212164,
0.0738483685540666));
#62015=CARTESIAN_POINT('Ctrl Pts',(0.00575623435121828,-0.0279779054956661,
0.0743074083721862));
#62016=CARTESIAN_POINT('Ctrl Pts',(0.00598037625292647,-0.0280826812445643,
0.0751677775536731));
#62017=CARTESIAN_POINT('Ctrl Pts',(0.006219576669604,-0.0281350691190143,
0.0755675389519453));
#62018=CARTESIAN_POINT('Ctrl Pts',(0.00688501715781157,-0.028239844867912,
0.0761750621069688));
#62019=CARTESIAN_POINT('Ctrl Pts',(0.00731030903013384,-0.0282922327423619,
0.0763814412976357));
#62020=CARTESIAN_POINT('Ctrl Pts',(0.00821272207368966,-0.0283970084912602,
0.0765234275937696));
#62021=CARTESIAN_POINT('Ctrl Pts',(0.0086881821973765,-0.0284493963657099,
0.0764583541632762));
#62022=CARTESIAN_POINT('Ctrl Pts',(0.00952801531425379,-0.0285541721146081,
0.0760670747619161));
#62023=CARTESIAN_POINT('Ctrl Pts',(0.00989050099342927,-0.028606559989058,
0.0757412514171181));
#62024=CARTESIAN_POINT('Ctrl Pts',(0.0103691372816368,-0.0287113357379557,
0.0749321489062033));
#62025=CARTESIAN_POINT('Ctrl Pts',(0.0104838416490414,-0.0287637236124047,
0.0744503508285196));
#62026=CARTESIAN_POINT('Ctrl Pts',(0.0104120206910918,-0.0288684993613048,
0.0734988043112581));
#62027=CARTESIAN_POINT('Ctrl Pts',(0.0102251237098014,-0.0289208872357529,
0.0730312547594835));
#62028=CARTESIAN_POINT('Ctrl Pts',(0.00960512622564884,-0.0290256629846524,
0.0722864423988114));
#62029=CARTESIAN_POINT('Ctrl Pts',(0.00917306831712077,-0.0290780508591023,
0.0720113501056385));
#62030=CARTESIAN_POINT('Ctrl Pts',(0.00821853372773986,-0.0291828266079989,
0.0717696960530468));
#62031=CARTESIAN_POINT('Ctrl Pts',(0.00769834660242158,-0.0292352144824501,
0.0718043795871957));
#62032=CARTESIAN_POINT('Ctrl Pts',(0.00677289295094829,-0.0293399902313469,
0.072185813448155));
#62033=CARTESIAN_POINT('Ctrl Pts',(0.00637042834480692,-0.029392378105796,
0.0725321781376852));
#62034=CARTESIAN_POINT('Ctrl Pts',(0.00585556439734561,-0.0294971538546968,
0.0734105506653613));
#62035=CARTESIAN_POINT('Ctrl Pts',(0.00574534815560973,-0.0295495417291453,
0.0739403889886591));
#62036=CARTESIAN_POINT('Ctrl Pts',(0.00588053728891275,-0.0296543174780434,
0.0749677637423445));
#62037=CARTESIAN_POINT('Ctrl Pts',(0.00612638441272354,-0.0297067053524937,
0.0754619701971907));
#62038=CARTESIAN_POINT('Ctrl Pts',(0.0068862121828339,-0.0298114811013907,
0.0761943297562885));
#62039=CARTESIAN_POINT('Ctrl Pts',(0.00739831304479771,-0.02986386897584,
0.0764293216352161));
#62040=CARTESIAN_POINT('Ctrl Pts',(0.00847024498270537,-0.0299686447247403,
0.0765167649077124));
#62041=CARTESIAN_POINT('Ctrl Pts',(0.00902628537726555,-0.0300210325991884,
0.0763678171248695));
#62042=CARTESIAN_POINT('Ctrl Pts',(0.00992055447858949,-0.0301258083480876,
0.0757326667816004));
#62043=CARTESIAN_POINT('Ctrl Pts',(0.0102545830055701,-0.0301781962225362,
0.0752479510576141));
#62044=CARTESIAN_POINT('Ctrl Pts',(0.0105208009285865,-0.0302829719714357,
0.0741604785186885));
#62045=CARTESIAN_POINT('Ctrl Pts',(0.0104505271100099,-0.0303353598458849,
0.073561995356696));
#62046=CARTESIAN_POINT('Ctrl Pts',(0.00991411670304272,-0.0304401355947827,
0.0725518154983641));
#62047=CARTESIAN_POINT('Ctrl Pts',(0.00944906750418523,-0.0304925234692313,
0.072145494478619));
#62048=CARTESIAN_POINT('Ctrl Pts',(0.00834579349582601,-0.0305972992181321,
0.0717572746685295));
#62049=CARTESIAN_POINT('Ctrl Pts',(0.00771250836259956,-0.0306496870925817,
0.0717790005685719));
#62050=CARTESIAN_POINT('Ctrl Pts',(0.00662086996932487,-0.0307544628414776,
0.0722706279495596));
#62051=CARTESIAN_POINT('Ctrl Pts',(0.00616934538289875,-0.0308068507159279,
0.0727396928462987));
#62052=CARTESIAN_POINT('Ctrl Pts',(0.00572829379585245,-0.0309116264648272,
0.0738846232116097));
#62053=CARTESIAN_POINT('Ctrl Pts',(0.00574362727005372,-0.030964014339277,
0.0745544281864965));
#62054=CARTESIAN_POINT('Ctrl Pts',(0.00621077743207889,-0.0310568507159276,
0.0755674191002066));
#62055=CARTESIAN_POINT('Ctrl Pts',(0.0065589500450449,-0.0310972992181319,
0.0759472268277333));
#62056=CARTESIAN_POINT('Ctrl Pts',(0.00742682523931609,-0.0311781962225358,
0.076428809978167));
#62057=CARTESIAN_POINT('Ctrl Pts',(0.00794469937310318,-0.0312186447247393,
0.0765285726773943));
#62058=CARTESIAN_POINT('Ctrl Pts',(0.00894927041430031,-0.0312995417291452,
0.0763879114871669));
#62059=CARTESIAN_POINT('Ctrl Pts',(0.00943299421279664,-0.031339990231348,
0.0761469018867863));
#62060=CARTESIAN_POINT('Ctrl Pts',(0.0101564533217469,-0.0314208872357532,
0.0754029570343451));
#62061=CARTESIAN_POINT('Ctrl Pts',(0.0103931454890576,-0.0314613357379553,
0.0749015233854856));
#62062=CARTESIAN_POINT('Ctrl Pts',(0.0104828841518005,-0.0315328667545812,
0.0739661159625376));
#62063=CARTESIAN_POINT('Ctrl Pts',(0.0104111042940494,-0.0315639492690025,
0.0735454439187662));
#62064=CARTESIAN_POINT('Ctrl Pts',(0.0102368137674672,-0.0315950317834238,
0.0731679328567764));
#62065=CARTESIAN_POINT('Ctrl Pts',(0.00815574178150025,-0.0204978184012171,
0.0766646002253042));
#62066=CARTESIAN_POINT('Ctrl Pts',(0.00842491138661719,-0.0205161211862624,
0.0766637306209027));
#62067=CARTESIAN_POINT('Ctrl Pts',(0.00869215025956532,-0.0205344239713078,
0.0766207916308805));
#62068=CARTESIAN_POINT('Ctrl Pts',(0.00980296761298115,-0.0206152267563535,
0.0762387652685163));
#62069=CARTESIAN_POINT('Ctrl Pts',(0.0104490879863571,-0.0206777267563525,
0.0754596377501276));
#62070=CARTESIAN_POINT('Ctrl Pts',(0.0107605546784065,-0.0208027267563538,
0.0737381396482117));
#62071=CARTESIAN_POINT('Ctrl Pts',(0.0104309111756661,-0.0208652267563538,
0.0728281886791785));
#62072=CARTESIAN_POINT('Ctrl Pts',(0.00916953442954738,-0.0209902267563526,
0.0717053258727286));
#62073=CARTESIAN_POINT('Ctrl Pts',(0.00826313610534649,-0.0210527267563532,
0.071503284888768));
#62074=CARTESIAN_POINT('Ctrl Pts',(0.00668440051922231,-0.0211777267563531,
0.0719245335753756));
#62075=CARTESIAN_POINT('Ctrl Pts',(0.0060317481102427,-0.0212402267563531,
0.0725351111673153));
#62076=CARTESIAN_POINT('Ctrl Pts',(0.00548408653655842,-0.0213652267563533,
0.0740216278732971));
#62077=CARTESIAN_POINT('Ctrl Pts',(0.00559006186519377,-0.0214277267563531,
0.0748774748910969));
#62078=CARTESIAN_POINT('Ctrl Pts',(0.00642784422772027,-0.0215527267563532,
0.0761681062534498));
#62079=CARTESIAN_POINT('Ctrl Pts',(0.0071463147509265,-0.0216152267563529,
0.0765916811367176));
#62080=CARTESIAN_POINT('Ctrl Pts',(0.00863687490376476,-0.0217402267563534,
0.076729531984443));
#62081=CARTESIAN_POINT('Ctrl Pts',(0.00939405041045344,-0.0218027267563532,
0.0764467767926095));
#62082=CARTESIAN_POINT('Ctrl Pts',(0.0104239081374065,-0.0219277267563531,
0.0754141936692029));
#62083=CARTESIAN_POINT('Ctrl Pts',(0.0106901560263932,-0.0219902267563532,
0.0746760822049604));
#62084=CARTESIAN_POINT('Ctrl Pts',(0.0105866970733117,-0.0221152267563531,
0.0732572024616046));
#62085=CARTESIAN_POINT('Ctrl Pts',(0.0102210256633657,-0.0221777267563529,
0.0725875487200949));
#62086=CARTESIAN_POINT('Ctrl Pts',(0.00912478396070292,-0.0223027267563535,
0.0717338709369279));
#62087=CARTESIAN_POINT('Ctrl Pts',(0.00840393535012082,-0.0223652267563527,
0.0715538671110964));
#62088=CARTESIAN_POINT('Ctrl Pts',(0.00706192316619711,-0.0224902267563536,
0.0717644503385637));
#62089=CARTESIAN_POINT('Ctrl Pts',(0.00644935225536766,-0.0225527267563534,
0.0721512045870529));
#62090=CARTESIAN_POINT('Ctrl Pts',(0.00568156547803287,-0.0226777267563529,
0.073236503285558));
#62091=CARTESIAN_POINT('Ctrl Pts',(0.00552930472474256,-0.0227402267563533,
0.0739271259238148));
#62092=CARTESIAN_POINT('Ctrl Pts',(0.00574579241785726,-0.022865226756353,
0.0752112025383953));
#62093=CARTESIAN_POINT('Ctrl Pts',(0.00611142407784697,-0.0229277267563529,
0.0757976905819331));
#62094=CARTESIAN_POINT('Ctrl Pts',(0.00713782884321568,-0.0230527267563535,
0.0765567333546231));
#62095=CARTESIAN_POINT('Ctrl Pts',(0.00779219947294575,-0.0231152267563532,
0.0767266731153024));
#62096=CARTESIAN_POINT('Ctrl Pts',(0.00903627529842336,-0.0232402267563531,
0.0765823954831315));
#62097=CARTESIAN_POINT('Ctrl Pts',(0.00962009289389314,-0.0233027267563532,
0.0762703943431882));
#62098=CARTESIAN_POINT('Ctrl Pts',(0.0104281726863687,-0.0234277267563531,
0.0753436508485646));
#62099=CARTESIAN_POINT('Ctrl Pts',(0.0106497998092528,-0.0234902267563532,
0.0747340104275962));
#62100=CARTESIAN_POINT('Ctrl Pts',(0.0106402475915358,-0.0236152267563531,
0.0735261129232099));
#62101=CARTESIAN_POINT('Ctrl Pts',(0.0104103399191558,-0.0236777267563534,
0.0729329580568231));
#62102=CARTESIAN_POINT('Ctrl Pts',(0.00962704552419596,-0.0238027267563529,
0.0720405600998036));
#62103=CARTESIAN_POINT('Ctrl Pts',(0.00907759547796414,-0.0238652267563534,
0.0717441147998457));
#62104=CARTESIAN_POINT('Ctrl Pts',(0.00792280197525823,-0.0239902267563529,
0.0715697576975107));
#62105=CARTESIAN_POINT('Ctrl Pts',(0.00732189290966092,-0.024052726756353,
0.0716914945714972));
#62106=CARTESIAN_POINT('Ctrl Pts',(0.00633576538864637,-0.0241777267563532,
0.0722817732256498));
#62107=CARTESIAN_POINT('Ctrl Pts',(0.00595351074227404,-0.0242402267563532,
0.0727474706965873));
#62108=CARTESIAN_POINT('Ctrl Pts',(0.00556232390452704,-0.0243652267563532,
0.0738092683440253));
#62109=CARTESIAN_POINT('Ctrl Pts',(0.0055538878949141,-0.0244277267563531,
0.0744015982618417));
#62110=CARTESIAN_POINT('Ctrl Pts',(0.00589936271740101,-0.0245527267563532,
0.0754613414480549));
#62111=CARTESIAN_POINT('Ctrl Pts',(0.00625147730318875,-0.0246152267563531,
0.075925717632976));
#62112=CARTESIAN_POINT('Ctrl Pts',(0.00715967514597056,-0.0247402267563532,
0.0765435739642516));
#62113=CARTESIAN_POINT('Ctrl Pts',(0.00771271308517418,-0.0248027267563532,
0.0766958326018746));
#62114=CARTESIAN_POINT('Ctrl Pts',(0.00879421128266716,-0.0249277267563531,
0.0766401337899241));
#62115=CARTESIAN_POINT('Ctrl Pts',(0.00931972040763655,-0.0249902267563527,
0.0764329755311924));
#62116=CARTESIAN_POINT('Ctrl Pts',(0.0101425971002925,-0.0251152267563537,
0.0757520711179273));
#62117=CARTESIAN_POINT('Ctrl Pts',(0.0104381935859063,-0.0251777267563533,
0.0752805635757531));
#62118=CARTESIAN_POINT('Ctrl Pts',(0.0106972561277655,-0.025302726756353,
0.0742591146587279));
#62119=CARTESIAN_POINT('Ctrl Pts',(0.0106606130882285,-0.0253652267563531,
0.0737118409737093));
#62120=CARTESIAN_POINT('Ctrl Pts',(0.0102802097636754,-0.0254902267563532,
0.0727438298599943));
#62121=CARTESIAN_POINT('Ctrl Pts',(0.00993781908349455,-0.0255527267563535,
0.0723251858403766));
#62122=CARTESIAN_POINT('Ctrl Pts',(0.00907974286877045,-0.0256777267563528,
0.0717611057473714));
#62123=CARTESIAN_POINT('Ctrl Pts',(0.00856623844841187,-0.0257402267563532,
0.0716165386221529));
#62124=CARTESIAN_POINT('Ctrl Pts',(0.00755239483066854,-0.0258652267563531,
0.0716424692265927));
#62125=CARTESIAN_POINT('Ctrl Pts',(0.00705420667293192,-0.0259277267563522,
0.0718124733178095));
#62126=CARTESIAN_POINT('Ctrl Pts',(0.0062418335830046,-0.0260527267563541,
0.0723989168441442));
#62127=CARTESIAN_POINT('Ctrl Pts',(0.00592906217181541,-0.0261152267563532,
0.072813831400163));
#62128=CARTESIAN_POINT('Ctrl Pts',(0.0054710080487956,-0.0262825025052516,
0.0740571267911857));
#62129=CARTESIAN_POINT('Ctrl Pts',(0.00559943784097573,-0.0263872782541498,
0.0749876671131497));
#62130=CARTESIAN_POINT('Ctrl Pts',(0.00661671847055469,-0.0265968297519482,
0.0763415199122333));
#62131=CARTESIAN_POINT('Ctrl Pts',(0.00749343156507586,-0.0267016055008472,
0.0767398321304675));
#62132=CARTESIAN_POINT('Ctrl Pts',(0.00921536343825145,-0.0269111569986424,
0.0765816707737669));
#62133=CARTESIAN_POINT('Ctrl Pts',(0.0100299612260055,-0.0270159327475413,
0.0760219906652354));
#62134=CARTESIAN_POINT('Ctrl Pts',(0.0107815284100618,-0.0272254842453399,
0.0744224932850827));
#62135=CARTESIAN_POINT('Ctrl Pts',(0.0106980646000727,-0.027330259994239,
0.0734101776580076));
#62136=CARTESIAN_POINT('Ctrl Pts',(0.0096415153281149,-0.0275398114920338,
0.0719430217203579));
#62137=CARTESIAN_POINT('Ctrl Pts',(0.00868406300525948,-0.0276445872409343,
0.0715231555974404));
#62138=CARTESIAN_POINT('Ctrl Pts',(0.00685097202868609,-0.0278541387387302,
0.0717847980264181));
#62139=CARTESIAN_POINT('Ctrl Pts',(0.00601829806137571,-0.0279589144876299,
0.0724691578228018));
#62140=CARTESIAN_POINT('Ctrl Pts',(0.00557900344885459,-0.028116078110977,
0.0738237074822833));
#62141=CARTESIAN_POINT('Ctrl Pts',(0.00556266611399862,-0.0281684659854268,
0.0743202779161881));
#62142=CARTESIAN_POINT('Ctrl Pts',(0.00580513362333878,-0.028273241734325,
0.0752509899827782));
#62143=CARTESIAN_POINT('Ctrl Pts',(0.00606389081609463,-0.028325629608775,
0.0756834354551811));
#62144=CARTESIAN_POINT('Ctrl Pts',(0.00678373702316377,-0.0284304053576727,
0.0763406290684345));
#62145=CARTESIAN_POINT('Ctrl Pts',(0.00724380031449291,-0.0284827932321226,
0.0765638816060427));
#62146=CARTESIAN_POINT('Ctrl Pts',(0.00821999370537458,-0.0285875689810209,
0.076717476553358));
#62147=CARTESIAN_POINT('Ctrl Pts',(0.00873432695186883,-0.0286399568554705,
0.0766470827871961));
#62148=CARTESIAN_POINT('Ctrl Pts',(0.00964282394666933,-0.0287447326043687,
0.0762238127909082));
#62149=CARTESIAN_POINT('Ctrl Pts',(0.010034946076139,-0.0287971204788187,
0.0758713504699588));
#62150=CARTESIAN_POINT('Ctrl Pts',(0.0105527151670457,-0.0289018962277164,
0.0749960965833477));
#62151=CARTESIAN_POINT('Ctrl Pts',(0.0106767976436514,-0.0289542841021654,
0.0744749071983615));
#62152=CARTESIAN_POINT('Ctrl Pts',(0.0105991046792403,-0.0290590598510655,
0.0734455632323137));
#62153=CARTESIAN_POINT('Ctrl Pts',(0.0103969271960863,-0.0291114477255137,
0.0729397873178239));
#62154=CARTESIAN_POINT('Ctrl Pts',(0.00972623936559113,-0.0292162234744131,
0.0721340798769493));
#62155=CARTESIAN_POINT('Ctrl Pts',(0.00925885685400708,-0.0292686113488629,
0.0718364963253867));
#62156=CARTESIAN_POINT('Ctrl Pts',(0.00822628051418617,-0.0293733870977596,
0.0715750848900085));
#62157=CARTESIAN_POINT('Ctrl Pts',(0.0076635634331514,-0.0294257749722108,
0.0716126041136615));
#62158=CARTESIAN_POINT('Ctrl Pts',(0.0066624456583287,-0.0295305507211076,
0.072025223608455));
#62159=CARTESIAN_POINT('Ctrl Pts',(0.00622707596660661,-0.0295829385955566,
0.0723999067130141));
#62160=CARTESIAN_POINT('Ctrl Pts',(0.00567011728088695,-0.0296877143444575,
0.0733500940605625));
#62161=CARTESIAN_POINT('Ctrl Pts',(0.00555088987441427,-0.0297401022189059,
0.0739232514114372));
#62162=CARTESIAN_POINT('Ctrl Pts',(0.00569713192996942,-0.029844877967804,
0.0750346232512706));
#62163=CARTESIAN_POINT('Ctrl Pts',(0.00596307925768723,-0.0298972658422544,
0.075569235509368));
#62164=CARTESIAN_POINT('Ctrl Pts',(0.00678502975218297,-0.0300020415911513,
0.0763614720206259));
#62165=CARTESIAN_POINT('Ctrl Pts',(0.00733899944542236,-0.0300544294656007,
0.0766156765899838));
#62166=CARTESIAN_POINT('Ctrl Pts',(0.00849857141829326,-0.0301592052145009,
0.076710269133052));
#62167=CARTESIAN_POINT('Ctrl Pts',(0.00910007309439272,-0.0302115930889491,
0.0765491435351497));
#62168=CARTESIAN_POINT('Ctrl Pts',(0.0100674567028369,-0.0303163688378483,
0.0758620639636131));
#62169=CARTESIAN_POINT('Ctrl Pts',(0.010428795053089,-0.0303687567122968,
0.0753377183886118));
#62170=CARTESIAN_POINT('Ctrl Pts',(0.0107167786752658,-0.0304735324611964,
0.0741613352314253));
#62171=CARTESIAN_POINT('Ctrl Pts',(0.0106407593427259,-0.0305259203356456,
0.0735139207115853));
#62172=CARTESIAN_POINT('Ctrl Pts',(0.0100604925814896,-0.0306306960845434,
0.072421149603779));
#62173=CARTESIAN_POINT('Ctrl Pts',(0.00955742144615823,-0.0306830839589921,
0.0719816082021071));
#62174=CARTESIAN_POINT('Ctrl Pts',(0.0083639449079113,-0.0307878597078928,
0.0715616479460749));
#62175=CARTESIAN_POINT('Ctrl Pts',(0.00767888304404099,-0.0308402475823424,
0.0715851501329989));
#62176=CARTESIAN_POINT('Ctrl Pts',(0.00649799343660759,-0.0309450233312383,
0.0721169724548543));
#62177=CARTESIAN_POINT('Ctrl Pts',(0.00600955267188516,-0.0309974112056886,
0.0726243876073294));
#62178=CARTESIAN_POINT('Ctrl Pts',(0.00553244116802694,-0.0311021869545879,
0.0738629262827373));
#62179=CARTESIAN_POINT('Ctrl Pts',(0.00554902829105363,-0.0311545748290377,
0.0745874938123549));
#62180=CARTESIAN_POINT('Ctrl Pts',(0.00605437216210567,-0.0312474112056882,
0.0756833058044895));
#62181=CARTESIAN_POINT('Ctrl Pts',(0.00643101100403122,-0.0312878597078925,
0.0760941662148802));
#62182=CARTESIAN_POINT('Ctrl Pts',(0.00736984276716638,-0.0313687567122965,
0.076615123100389));
#62183=CARTESIAN_POINT('Ctrl Pts',(0.00793005774889972,-0.0314092052144999,
0.0767230422936426));
#62184=CARTESIAN_POINT('Ctrl Pts',(0.00901676146854406,-0.0314901022189058,
0.076570880791508));
#62185=CARTESIAN_POINT('Ctrl Pts',(0.00954003401926395,-0.0315305507211086,
0.0763101664980802));
#62186=CARTESIAN_POINT('Ctrl Pts',(0.0103226423888721,-0.0316114477255139,
0.075505397492003));
#62187=CARTESIAN_POINT('Ctrl Pts',(0.0105786862604142,-0.0316518962277159,
0.0749629671520629));
#62188=CARTESIAN_POINT('Ctrl Pts',(0.0106757618624369,-0.0317234272443419,
0.0739510817958126));
#62189=CARTESIAN_POINT('Ctrl Pts',(0.0105981133585333,-0.0317545097587632,
0.0734960160453883));
#62190=CARTESIAN_POINT('Ctrl Pts',(0.0104095730206495,-0.0317855922731845,
0.0730876400735085));
#62191=CARTESIAN_POINT('Ctrl Pts',(0.00815574178150025,-0.0209166974216957,
0.0766646002253042));
#62192=CARTESIAN_POINT('Ctrl Pts',(0.00842491138661719,-0.020935000206741,
0.0766637306209027));
#62193=CARTESIAN_POINT('Ctrl Pts',(0.00869215025956532,-0.0209533029917864,
0.0766207916308805));
#62194=CARTESIAN_POINT('Ctrl Pts',(0.00980296761298115,-0.0210341057768321,
0.0762387652685163));
#62195=CARTESIAN_POINT('Ctrl Pts',(0.0104490879863571,-0.0210966057768311,
0.0754596377501276));
#62196=CARTESIAN_POINT('Ctrl Pts',(0.0107605546784065,-0.0212216057768325,
0.0737381396482117));
#62197=CARTESIAN_POINT('Ctrl Pts',(0.0104309111756661,-0.0212841057768323,
0.0728281886791785));
#62198=CARTESIAN_POINT('Ctrl Pts',(0.00916953442954738,-0.0214091057768312,
0.0717053258727286));
#62199=CARTESIAN_POINT('Ctrl Pts',(0.00826313610534649,-0.0214716057768319,
0.071503284888768));
#62200=CARTESIAN_POINT('Ctrl Pts',(0.00668440051922231,-0.0215966057768317,
0.0719245335753756));
#62201=CARTESIAN_POINT('Ctrl Pts',(0.0060317481102427,-0.0216591057768317,
0.0725351111673153));
#62202=CARTESIAN_POINT('Ctrl Pts',(0.00548408653655842,-0.0217841057768319,
0.0740216278732971));
#62203=CARTESIAN_POINT('Ctrl Pts',(0.00559006186519377,-0.0218466057768317,
0.0748774748910969));
#62204=CARTESIAN_POINT('Ctrl Pts',(0.00642784422772027,-0.0219716057768319,
0.0761681062534498));
#62205=CARTESIAN_POINT('Ctrl Pts',(0.0071463147509265,-0.0220341057768316,
0.0765916811367176));
#62206=CARTESIAN_POINT('Ctrl Pts',(0.00863687490376476,-0.0221591057768321,
0.076729531984443));
#62207=CARTESIAN_POINT('Ctrl Pts',(0.00939405041045344,-0.0222216057768319,
0.0764467767926095));
#62208=CARTESIAN_POINT('Ctrl Pts',(0.0104239081374065,-0.0223466057768317,
0.0754141936692029));
#62209=CARTESIAN_POINT('Ctrl Pts',(0.0106901560263932,-0.0224091057768319,
0.0746760822049604));
#62210=CARTESIAN_POINT('Ctrl Pts',(0.0105866970733117,-0.0225341057768317,
0.0732572024616046));
#62211=CARTESIAN_POINT('Ctrl Pts',(0.0102210256633657,-0.0225966057768315,
0.0725875487200949));
#62212=CARTESIAN_POINT('Ctrl Pts',(0.00912478396070292,-0.0227216057768321,
0.0717338709369279));
#62213=CARTESIAN_POINT('Ctrl Pts',(0.00840393535012082,-0.0227841057768314,
0.0715538671110964));
#62214=CARTESIAN_POINT('Ctrl Pts',(0.00706192316619711,-0.0229091057768322,
0.0717644503385637));
#62215=CARTESIAN_POINT('Ctrl Pts',(0.00644935225536766,-0.0229716057768321,
0.0721512045870529));
#62216=CARTESIAN_POINT('Ctrl Pts',(0.00568156547803287,-0.0230966057768316,
0.073236503285558));
#62217=CARTESIAN_POINT('Ctrl Pts',(0.00552930472474256,-0.023159105776832,
0.0739271259238148));
#62218=CARTESIAN_POINT('Ctrl Pts',(0.00574579241785726,-0.0232841057768316,
0.0752112025383953));
#62219=CARTESIAN_POINT('Ctrl Pts',(0.00611142407784697,-0.0233466057768315,
0.0757976905819331));
#62220=CARTESIAN_POINT('Ctrl Pts',(0.00713782884321568,-0.0234716057768321,
0.0765567333546231));
#62221=CARTESIAN_POINT('Ctrl Pts',(0.00779219947294575,-0.0235341057768318,
0.0767266731153024));
#62222=CARTESIAN_POINT('Ctrl Pts',(0.00903627529842336,-0.0236591057768317,
0.0765823954831315));
#62223=CARTESIAN_POINT('Ctrl Pts',(0.00962009289389314,-0.0237216057768318,
0.0762703943431882));
#62224=CARTESIAN_POINT('Ctrl Pts',(0.0104281726863687,-0.0238466057768318,
0.0753436508485646));
#62225=CARTESIAN_POINT('Ctrl Pts',(0.0106497998092528,-0.0239091057768318,
0.0747340104275962));
#62226=CARTESIAN_POINT('Ctrl Pts',(0.0106402475915358,-0.0240341057768317,
0.0735261129232099));
#62227=CARTESIAN_POINT('Ctrl Pts',(0.0104103399191558,-0.0240966057768321,
0.0729329580568231));
#62228=CARTESIAN_POINT('Ctrl Pts',(0.00962704552419596,-0.0242216057768316,
0.0720405600998036));
#62229=CARTESIAN_POINT('Ctrl Pts',(0.00907759547796414,-0.0242841057768321,
0.0717441147998457));
#62230=CARTESIAN_POINT('Ctrl Pts',(0.00792280197525823,-0.0244091057768316,
0.0715697576975107));
#62231=CARTESIAN_POINT('Ctrl Pts',(0.00732189290966092,-0.0244716057768317,
0.0716914945714972));
#62232=CARTESIAN_POINT('Ctrl Pts',(0.00633576538864637,-0.0245966057768319,
0.0722817732256498));
#62233=CARTESIAN_POINT('Ctrl Pts',(0.00595351074227404,-0.0246591057768318,
0.0727474706965873));
#62234=CARTESIAN_POINT('Ctrl Pts',(0.00556232390452704,-0.0247841057768317,
0.0738092683440253));
#62235=CARTESIAN_POINT('Ctrl Pts',(0.0055538878949141,-0.0248466057768317,
0.0744015982618417));
#62236=CARTESIAN_POINT('Ctrl Pts',(0.00589936271740101,-0.0249716057768318,
0.0754613414480549));
#62237=CARTESIAN_POINT('Ctrl Pts',(0.00625147730318875,-0.0250341057768317,
0.075925717632976));
#62238=CARTESIAN_POINT('Ctrl Pts',(0.00715967514597056,-0.0251591057768318,
0.0765435739642516));
#62239=CARTESIAN_POINT('Ctrl Pts',(0.00771271308517418,-0.0252216057768319,
0.0766958326018746));
#62240=CARTESIAN_POINT('Ctrl Pts',(0.00879421128266716,-0.0253466057768317,
0.0766401337899241));
#62241=CARTESIAN_POINT('Ctrl Pts',(0.00931972040763655,-0.0254091057768313,
0.0764329755311924));
#62242=CARTESIAN_POINT('Ctrl Pts',(0.0101425971002925,-0.0255341057768323,
0.0757520711179273));
#62243=CARTESIAN_POINT('Ctrl Pts',(0.0104381935859063,-0.025596605776832,
0.0752805635757531));
#62244=CARTESIAN_POINT('Ctrl Pts',(0.0106972561277655,-0.0257216057768316,
0.0742591146587279));
#62245=CARTESIAN_POINT('Ctrl Pts',(0.0106606130882285,-0.0257841057768317,
0.0737118409737093));
#62246=CARTESIAN_POINT('Ctrl Pts',(0.0102802097636754,-0.0259091057768319,
0.0727438298599943));
#62247=CARTESIAN_POINT('Ctrl Pts',(0.00993781908349455,-0.0259716057768321,
0.0723251858403766));
#62248=CARTESIAN_POINT('Ctrl Pts',(0.00907974286877045,-0.0260966057768315,
0.0717611057473714));
#62249=CARTESIAN_POINT('Ctrl Pts',(0.00856623844841187,-0.0261591057768319,
0.0716165386221529));
#62250=CARTESIAN_POINT('Ctrl Pts',(0.00755239483066854,-0.0262841057768317,
0.0716424692265927));
#62251=CARTESIAN_POINT('Ctrl Pts',(0.00705420667293192,-0.0263466057768309,
0.0718124733178095));
#62252=CARTESIAN_POINT('Ctrl Pts',(0.0062418335830046,-0.0264716057768327,
0.0723989168441442));
#62253=CARTESIAN_POINT('Ctrl Pts',(0.00592906217181541,-0.0265341057768319,
0.072813831400163));
#62254=CARTESIAN_POINT('Ctrl Pts',(0.0054710080487956,-0.0267013815257303,
0.0740571267911857));
#62255=CARTESIAN_POINT('Ctrl Pts',(0.00559943784097573,-0.0268061572746284,
0.0749876671131497));
#62256=CARTESIAN_POINT('Ctrl Pts',(0.00661671847055469,-0.0270157087724267,
0.0763415199122333));
#62257=CARTESIAN_POINT('Ctrl Pts',(0.00749343156507586,-0.0271204845213259,
0.0767398321304675));
#62258=CARTESIAN_POINT('Ctrl Pts',(0.00921536343825145,-0.027330036019121,
0.0765816707737669));
#62259=CARTESIAN_POINT('Ctrl Pts',(0.0100299612260055,-0.0274348117680204,
0.0760219906652354));
#62260=CARTESIAN_POINT('Ctrl Pts',(0.0107815284100618,-0.027644363265818,
0.0744224932850827));
#62261=CARTESIAN_POINT('Ctrl Pts',(0.0106980646000727,-0.0277491390147176,
0.0734101776580076));
#62262=CARTESIAN_POINT('Ctrl Pts',(0.0096415153281149,-0.0279586905125125,
0.0719430217203579));
#62263=CARTESIAN_POINT('Ctrl Pts',(0.00868406300525948,-0.028063466261413,
0.0715231555974404));
#62264=CARTESIAN_POINT('Ctrl Pts',(0.00685097202868609,-0.0282730177592087,
0.0717847980264181));
#62265=CARTESIAN_POINT('Ctrl Pts',(0.00601829806137571,-0.0283777935081086,
0.0724691578228018));
#62266=CARTESIAN_POINT('Ctrl Pts',(0.00557900344885459,-0.0285349571314557,
0.0738237074822833));
#62267=CARTESIAN_POINT('Ctrl Pts',(0.00556266611399862,-0.0285873450059055,
0.0743202779161881));
#62268=CARTESIAN_POINT('Ctrl Pts',(0.00580513362333878,-0.0286921207548037,
0.0752509899827782));
#62269=CARTESIAN_POINT('Ctrl Pts',(0.00606389081609463,-0.0287445086292537,
0.0756834354551811));
#62270=CARTESIAN_POINT('Ctrl Pts',(0.00678373702316377,-0.0288492843781513,
0.0763406290684345));
#62271=CARTESIAN_POINT('Ctrl Pts',(0.00724380031449291,-0.0289016722526012,
0.0765638816060427));
#62272=CARTESIAN_POINT('Ctrl Pts',(0.00821999370537458,-0.0290064480014996,
0.076717476553358));
#62273=CARTESIAN_POINT('Ctrl Pts',(0.00873432695186883,-0.0290588358759492,
0.0766470827871961));
#62274=CARTESIAN_POINT('Ctrl Pts',(0.00964282394666933,-0.0291636116248473,
0.0762238127909082));
#62275=CARTESIAN_POINT('Ctrl Pts',(0.010034946076139,-0.0292159994992974,
0.0758713504699588));
#62276=CARTESIAN_POINT('Ctrl Pts',(0.0105527151670457,-0.029320775248195,
0.0749960965833477));
#62277=CARTESIAN_POINT('Ctrl Pts',(0.0106767976436514,-0.029373163122644,
0.0744749071983615));
#62278=CARTESIAN_POINT('Ctrl Pts',(0.0105991046792403,-0.0294779388715441,
0.0734455632323137));
#62279=CARTESIAN_POINT('Ctrl Pts',(0.0103969271960863,-0.0295303267459923,
0.0729397873178239));
#62280=CARTESIAN_POINT('Ctrl Pts',(0.00972623936559113,-0.0296351024948917,
0.0721340798769493));
#62281=CARTESIAN_POINT('Ctrl Pts',(0.00925885685400708,-0.0296874903693416,
0.0718364963253867));
#62282=CARTESIAN_POINT('Ctrl Pts',(0.00822628051418617,-0.0297922661182383,
0.0715750848900085));
#62283=CARTESIAN_POINT('Ctrl Pts',(0.0076635634331514,-0.0298446539926894,
0.0716126041136615));
#62284=CARTESIAN_POINT('Ctrl Pts',(0.0066624456583287,-0.0299494297415862,
0.072025223608455));
#62285=CARTESIAN_POINT('Ctrl Pts',(0.00622707596660661,-0.0300018176160353,
0.0723999067130141));
#62286=CARTESIAN_POINT('Ctrl Pts',(0.00567011728088695,-0.0301065933649361,
0.0733500940605625));
#62287=CARTESIAN_POINT('Ctrl Pts',(0.00555088987441427,-0.0301589812393846,
0.0739232514114372));
#62288=CARTESIAN_POINT('Ctrl Pts',(0.00569713192996942,-0.0302637569882826,
0.0750346232512706));
#62289=CARTESIAN_POINT('Ctrl Pts',(0.00596307925768723,-0.0303161448627331,
0.075569235509368));
#62290=CARTESIAN_POINT('Ctrl Pts',(0.00678502975218297,-0.03042092061163,
0.0763614720206259));
#62291=CARTESIAN_POINT('Ctrl Pts',(0.00733899944542236,-0.0304733084860793,
0.0766156765899838));
#62292=CARTESIAN_POINT('Ctrl Pts',(0.00849857141829326,-0.0305780842349796,
0.076710269133052));
#62293=CARTESIAN_POINT('Ctrl Pts',(0.00910007309439272,-0.0306304721094278,
0.0765491435351497));
#62294=CARTESIAN_POINT('Ctrl Pts',(0.0100674567028369,-0.030735247858327,
0.0758620639636131));
#62295=CARTESIAN_POINT('Ctrl Pts',(0.010428795053089,-0.0307876357327754,
0.0753377183886118));
#62296=CARTESIAN_POINT('Ctrl Pts',(0.0107167786752658,-0.030892411481675,
0.0741613352314253));
#62297=CARTESIAN_POINT('Ctrl Pts',(0.0106407593427259,-0.0309447993561243,
0.0735139207115853));
#62298=CARTESIAN_POINT('Ctrl Pts',(0.0100604925814896,-0.031049575105022,
0.072421149603779));
#62299=CARTESIAN_POINT('Ctrl Pts',(0.00955742144615823,-0.0311019629794706,
0.0719816082021071));
#62300=CARTESIAN_POINT('Ctrl Pts',(0.0083639449079113,-0.0312067387283715,
0.0715616479460749));
#62301=CARTESIAN_POINT('Ctrl Pts',(0.00767888304404099,-0.031259126602821,
0.0715851501329989));
#62302=CARTESIAN_POINT('Ctrl Pts',(0.00649799343660759,-0.0313639023517169,
0.0721169724548543));
#62303=CARTESIAN_POINT('Ctrl Pts',(0.00600955267188516,-0.0314162902261672,
0.0726243876073294));
#62304=CARTESIAN_POINT('Ctrl Pts',(0.00553244116802694,-0.0315210659750665,
0.0738629262827373));
#62305=CARTESIAN_POINT('Ctrl Pts',(0.00554902829105363,-0.0315734538495163,
0.0745874938123549));
#62306=CARTESIAN_POINT('Ctrl Pts',(0.00605437216210567,-0.0316662902261669,
0.0756833058044895));
#62307=CARTESIAN_POINT('Ctrl Pts',(0.00643101100403122,-0.0317067387283712,
0.0760941662148802));
#62308=CARTESIAN_POINT('Ctrl Pts',(0.00736984276716638,-0.0317876357327751,
0.076615123100389));
#62309=CARTESIAN_POINT('Ctrl Pts',(0.00793005774889972,-0.0318280842349786,
0.0767230422936426));
#62310=CARTESIAN_POINT('Ctrl Pts',(0.00901676146854406,-0.0319089812393844,
0.076570880791508));
#62311=CARTESIAN_POINT('Ctrl Pts',(0.00954003401926395,-0.0319494297415873,
0.0763101664980802));
#62312=CARTESIAN_POINT('Ctrl Pts',(0.0103226423888721,-0.0320303267459926,
0.075505397492003));
#62313=CARTESIAN_POINT('Ctrl Pts',(0.0105786862604142,-0.0320707752481946,
0.0749629671520629));
#62314=CARTESIAN_POINT('Ctrl Pts',(0.0106757618624369,-0.0321423062648206,
0.0739510817958126));
#62315=CARTESIAN_POINT('Ctrl Pts',(0.0105981133585333,-0.0321733887792418,
0.0734960160453883));
#62316=CARTESIAN_POINT('Ctrl Pts',(0.0104095730206495,-0.0322044712936632,
0.0730876400735085));
#62317=CARTESIAN_POINT('Ctrl Pts',(0.00815332628724061,-0.0211072579114564,
0.0764745476396777));
#62318=CARTESIAN_POINT('Ctrl Pts',(0.00840215214987724,-0.0211255606965017,
0.0764737437596658));
#62319=CARTESIAN_POINT('Ctrl Pts',(0.00864919320439181,-0.0211438634815471,
0.0764340500831514));
#62320=CARTESIAN_POINT('Ctrl Pts',(0.00967605537954476,-0.0212246662665928,
0.0760808971366146));
#62321=CARTESIAN_POINT('Ctrl Pts',(0.0102733422062002,-0.0212871662665918,
0.0753606557973937));
#62322=CARTESIAN_POINT('Ctrl Pts',(0.0105612683570671,-0.0214121662665932,
0.0737692679062889));
#62323=CARTESIAN_POINT('Ctrl Pts',(0.0102565391923597,-0.021474666266593,
0.0729280907060315));
#62324=CARTESIAN_POINT('Ctrl Pts',(0.00909049684955361,-0.0215996662665919,
0.0718900934688763));
#62325=CARTESIAN_POINT('Ctrl Pts',(0.00825260378650262,-0.0216621662665925,
0.0717033226702191));
#62326=CARTESIAN_POINT('Ctrl Pts',(0.00679318847130807,-0.0217871662665924,
0.0720927335317618));
#62327=CARTESIAN_POINT('Ctrl Pts',(0.00618986329796383,-0.0218496662665923,
0.0726571638876892));
#62328=CARTESIAN_POINT('Ctrl Pts',(0.00568359379013531,-0.0219746662665926,
0.0740313301927182));
#62329=CARTESIAN_POINT('Ctrl Pts',(0.00578155954133694,-0.0220371662665924,
0.0748224925990252));
#62330=CARTESIAN_POINT('Ctrl Pts',(0.00655602261255478,-0.0221621662665925,
0.076015578504634));
#62331=CARTESIAN_POINT('Ctrl Pts',(0.00722019139059382,-0.0222246662665922,
0.0764071397497255));
#62332=CARTESIAN_POINT('Ctrl Pts',(0.00859809554021233,-0.0223496662665927,
0.0765345718796849));
#62333=CARTESIAN_POINT('Ctrl Pts',(0.00929804399292574,-0.0224121662665926,
0.0762731872241167));
#62334=CARTESIAN_POINT('Ctrl Pts',(0.010250065441227,-0.0225371662665923,
0.0753186463638511));
#62335=CARTESIAN_POINT('Ctrl Pts',(0.0104961904099933,-0.0225996662665926,
0.0746363211000744));
#62336=CARTESIAN_POINT('Ctrl Pts',(0.0104005508475817,-0.0227246662665924,
0.0733246797802278));
#62337=CARTESIAN_POINT('Ctrl Pts',(0.0100625167520088,-0.0227871662665921,
0.0727056382289851));
#62338=CARTESIAN_POINT('Ctrl Pts',(0.00904912860513842,-0.0229121662665928,
0.0719164811073332));
#62339=CARTESIAN_POINT('Ctrl Pts',(0.00838276147471677,-0.0229746662665921,
0.0717500819062757));
#62340=CARTESIAN_POINT('Ctrl Pts',(0.00714217809165384,-0.0230996662665929,
0.0719447493287309));
#62341=CARTESIAN_POINT('Ctrl Pts',(0.0065759050711654,-0.0231621662665927,
0.0723022728294504));
#62342=CARTESIAN_POINT('Ctrl Pts',(0.00586614734384593,-0.0232871662665922,
0.0733055450405034));
#62343=CARTESIAN_POINT('Ctrl Pts',(0.00572539440382979,-0.0233496662665926,
0.073943970666777));
#62344=CARTESIAN_POINT('Ctrl Pts',(0.00592552003453053,-0.0234746662665924,
0.0751309972301058));
#62345=CARTESIAN_POINT('Ctrl Pts',(0.00626351738443437,-0.0235371662665921,
0.0756731587170833));
#62346=CARTESIAN_POINT('Ctrl Pts',(0.00721234684475271,-0.0236621662665928,
0.0763748333085017));
#62347=CARTESIAN_POINT('Ctrl Pts',(0.00781726037633776,-0.0237246662665926,
0.0765319290828517));
#62348=CARTESIAN_POINT('Ctrl Pts',(0.00896730939589689,-0.0238496662665925,
0.076398555902516));
#62349=CARTESIAN_POINT('Ctrl Pts',(0.00950700226631619,-0.0239121662665925,
0.0761101356971356));
#62350=CARTESIAN_POINT('Ctrl Pts',(0.010254007677104,-0.0240371662665925,
0.0752534351443655));
#62351=CARTESIAN_POINT('Ctrl Pts',(0.0104588843013103,-0.0240996662665926,
0.0746898711283627));
#62352=CARTESIAN_POINT('Ctrl Pts',(0.0104500540367917,-0.0242246662665924,
0.0735732660853268));
#62353=CARTESIAN_POINT('Ctrl Pts',(0.0102375227040588,-0.0242871662665928,
0.0730249416515866));
#62354=CARTESIAN_POINT('Ctrl Pts',(0.00951342941930744,-0.0244121662665922,
0.0721999908129729));
#62355=CARTESIAN_POINT('Ctrl Pts',(0.00900550661104702,-0.0244746662665927,
0.0719259507427556));
#62356=CARTESIAN_POINT('Ctrl Pts',(0.00793799198823834,-0.0245996662665922,
0.0717647714878526));
#62357=CARTESIAN_POINT('Ctrl Pts',(0.0073824994148905,-0.0246621662665923,
0.071877307532445));
#62358=CARTESIAN_POINT('Ctrl Pts',(0.00647090305920422,-0.0247871662665926,
0.0724229731370429));
#62359=CARTESIAN_POINT('Ctrl Pts',(0.0061175390822829,-0.0248496662665925,
0.0728534733596938));
#62360=CARTESIAN_POINT('Ctrl Pts',(0.0057559180058162,-0.0249746662665924,
0.0738350207207137));
#62361=CARTESIAN_POINT('Ctrl Pts',(0.00574811958679247,-0.0250371662665924,
0.0743825825552014));
#62362=CARTESIAN_POINT('Ctrl Pts',(0.00606748354576255,-0.0251621662665925,
0.075362230730441));
#62363=CARTESIAN_POINT('Ctrl Pts',(0.00639298543709791,-0.0252246662665924,
0.0757915095294001));
#62364=CARTESIAN_POINT('Ctrl Pts',(0.00723254201175921,-0.0253496662665925,
0.0763626685001477));
#62365=CARTESIAN_POINT('Ctrl Pts',(0.00774378154132399,-0.0254121662665926,
0.0765034194843978));
#62366=CARTESIAN_POINT('Ctrl Pts',(0.00874354049187196,-0.0255371662665924,
0.0764519303687327));
#62367=CARTESIAN_POINT('Ctrl Pts',(0.00922933182513614,-0.025599666266592,
0.0762604290571012));
#62368=CARTESIAN_POINT('Ctrl Pts',(0.00999001579168093,-0.0257246662665929,
0.0756309871558503));
#62369=CARTESIAN_POINT('Ctrl Pts',(0.0102632712006387,-0.0257871662665926,
0.0751951159850686));
#62370=CARTESIAN_POINT('Ctrl Pts',(0.0105027538882435,-0.0259121662665923,
0.0742508678118485));
#62371=CARTESIAN_POINT('Ctrl Pts',(0.0104688803165286,-0.0259746662665924,
0.0737449568761991));
#62372=CARTESIAN_POINT('Ctrl Pts',(0.0101172277391856,-0.0260996662665926,
0.0728501076962283));
#62373=CARTESIAN_POINT('Ctrl Pts',(0.00980071482414927,-0.0261621662665928,
0.0724631046418761));
#62374=CARTESIAN_POINT('Ctrl Pts',(0.00900749170282425,-0.0262871662665921,
0.0719416575205446));
#62375=CARTESIAN_POINT('Ctrl Pts',(0.00853279776289023,-0.0263496662665926,
0.0718080167269426));
#62376=CARTESIAN_POINT('Ctrl Pts',(0.0075955800831525,-0.0264746662665923,
0.0718319875055733));
#62377=CARTESIAN_POINT('Ctrl Pts',(0.0071350448081896,-0.0265371662665915,
0.0719891427483816));
#62378=CARTESIAN_POINT('Ctrl Pts',(0.0063840705858361,-0.0266621662665934,
0.0725312630827505));
#62379=CARTESIAN_POINT('Ctrl Pts',(0.00609493832603504,-0.0267246662665926,
0.0729148185450287));
#62380=CARTESIAN_POINT('Ctrl Pts',(0.00567150376979967,-0.0268919420154909,
0.0740641461150897));
#62381=CARTESIAN_POINT('Ctrl Pts',(0.00579022688422278,-0.0269967177643891,
0.0749243565323479));
#62382=CARTESIAN_POINT('Ctrl Pts',(0.00673062180767083,-0.0272062692621875,
0.0761758856211119));
#62383=CARTESIAN_POINT('Ctrl Pts',(0.00754107324008372,-0.0273110450110865,
0.076544093544357));
#62384=CARTESIAN_POINT('Ctrl Pts',(0.00913286211817163,-0.0275205965088817,
0.0763978859664261));
#62385=CARTESIAN_POINT('Ctrl Pts',(0.00988589289648584,-0.0276253722577802,
0.0758805062803154));
#62386=CARTESIAN_POINT('Ctrl Pts',(0.0105806569015859,-0.0278349237555796,
0.0744018983400594));
#62387=CARTESIAN_POINT('Ctrl Pts',(0.0105035012565028,-0.0279396995044774,
0.0734660931660017));
#62388=CARTESIAN_POINT('Ctrl Pts',(0.00952680560062186,-0.028149251002274,
0.072109824349359));
#62389=CARTESIAN_POINT('Ctrl Pts',(0.00864171718187381,-0.0282540267511745,
0.0717216915578374));
#62390=CARTESIAN_POINT('Ctrl Pts',(0.00694717056566465,-0.0284635782489686,
0.0719635591456149));
#62391=CARTESIAN_POINT('Ctrl Pts',(0.0061774297989796,-0.0285683539978693,
0.0725961952733644));
#62392=CARTESIAN_POINT('Ctrl Pts',(0.00577133691614923,-0.0287255176212164,
0.0738483685540666));
#62393=CARTESIAN_POINT('Ctrl Pts',(0.00575623435121828,-0.0287779054956661,
0.0743074083721862));
#62394=CARTESIAN_POINT('Ctrl Pts',(0.00598037625292647,-0.0288826812445643,
0.0751677775536731));
#62395=CARTESIAN_POINT('Ctrl Pts',(0.006219576669604,-0.0289350691190143,
0.0755675389519453));
#62396=CARTESIAN_POINT('Ctrl Pts',(0.00688501715781157,-0.0290398448679119,
0.0761750621069688));
#62397=CARTESIAN_POINT('Ctrl Pts',(0.00731030903013384,-0.0290922327423619,
0.0763814412976357));
#62398=CARTESIAN_POINT('Ctrl Pts',(0.00821272207368966,-0.0291970084912602,
0.0765234275937696));
#62399=CARTESIAN_POINT('Ctrl Pts',(0.0086881821973765,-0.0292493963657099,
0.0764583541632762));
#62400=CARTESIAN_POINT('Ctrl Pts',(0.00952801531425379,-0.0293541721146081,
0.0760670747619161));
#62401=CARTESIAN_POINT('Ctrl Pts',(0.00989050099342927,-0.029406559989058,
0.0757412514171181));
#62402=CARTESIAN_POINT('Ctrl Pts',(0.0103691372816368,-0.0295113357379557,
0.0749321489062033));
#62403=CARTESIAN_POINT('Ctrl Pts',(0.0104838416490414,-0.0295637236124048,
0.0744503508285196));
#62404=CARTESIAN_POINT('Ctrl Pts',(0.0104120206910918,-0.0296684993613048,
0.0734988043112581));
#62405=CARTESIAN_POINT('Ctrl Pts',(0.0102251237098014,-0.0297208872357529,
0.0730312547594835));
#62406=CARTESIAN_POINT('Ctrl Pts',(0.00960512622564884,-0.0298256629846524,
0.0722864423988114));
#62407=CARTESIAN_POINT('Ctrl Pts',(0.00917306831712077,-0.0298780508591023,
0.0720113501056385));
#62408=CARTESIAN_POINT('Ctrl Pts',(0.00821853372773986,-0.0299828266079989,
0.0717696960530468));
#62409=CARTESIAN_POINT('Ctrl Pts',(0.00769834660242158,-0.03003521448245,
0.0718043795871957));
#62410=CARTESIAN_POINT('Ctrl Pts',(0.00677289295094829,-0.030139990231347,
0.072185813448155));
#62411=CARTESIAN_POINT('Ctrl Pts',(0.00637042834480692,-0.030192378105796,
0.0725321781376852));
#62412=CARTESIAN_POINT('Ctrl Pts',(0.00585556439734561,-0.0302971538546968,
0.0734105506653613));
#62413=CARTESIAN_POINT('Ctrl Pts',(0.00574534815560973,-0.0303495417291453,
0.0739403889886591));
#62414=CARTESIAN_POINT('Ctrl Pts',(0.00588053728891275,-0.0304543174780433,
0.0749677637423445));
#62415=CARTESIAN_POINT('Ctrl Pts',(0.00612638441272354,-0.0305067053524937,
0.0754619701971907));
#62416=CARTESIAN_POINT('Ctrl Pts',(0.0068862121828339,-0.0306114811013907,
0.0761943297562885));
#62417=CARTESIAN_POINT('Ctrl Pts',(0.00739831304479771,-0.03066386897584,
0.0764293216352161));
#62418=CARTESIAN_POINT('Ctrl Pts',(0.00847024498270537,-0.0307686447247403,
0.0765167649077124));
#62419=CARTESIAN_POINT('Ctrl Pts',(0.00902628537726555,-0.0308210325991885,
0.0763678171248695));
#62420=CARTESIAN_POINT('Ctrl Pts',(0.00992055447858949,-0.0309258083480876,
0.0757326667816004));
#62421=CARTESIAN_POINT('Ctrl Pts',(0.0102545830055701,-0.0309781962225361,
0.0752479510576141));
#62422=CARTESIAN_POINT('Ctrl Pts',(0.0105208009285865,-0.0310829719714357,
0.0741604785186885));
#62423=CARTESIAN_POINT('Ctrl Pts',(0.0104505271100099,-0.031135359845885,
0.073561995356696));
#62424=CARTESIAN_POINT('Ctrl Pts',(0.00991411670304271,-0.0312401355947827,
0.0725518154983641));
#62425=CARTESIAN_POINT('Ctrl Pts',(0.00944906750418523,-0.0312925234692314,
0.072145494478619));
#62426=CARTESIAN_POINT('Ctrl Pts',(0.00834579349582601,-0.0313972992181321,
0.0717572746685295));
#62427=CARTESIAN_POINT('Ctrl Pts',(0.00771250836259956,-0.0314496870925817,
0.0717790005685719));
#62428=CARTESIAN_POINT('Ctrl Pts',(0.00662086996932487,-0.0315544628414776,
0.0722706279495596));
#62429=CARTESIAN_POINT('Ctrl Pts',(0.00616934538289875,-0.0316068507159279,
0.0727396928462987));
#62430=CARTESIAN_POINT('Ctrl Pts',(0.00572829379585245,-0.0317116264648272,
0.0738846232116097));
#62431=CARTESIAN_POINT('Ctrl Pts',(0.00574362727005372,-0.031764014339277,
0.0745544281864965));
#62432=CARTESIAN_POINT('Ctrl Pts',(0.00621077743207889,-0.0318568507159276,
0.0755674191002066));
#62433=CARTESIAN_POINT('Ctrl Pts',(0.0065589500450449,-0.0318972992181318,
0.0759472268277333));
#62434=CARTESIAN_POINT('Ctrl Pts',(0.00742682523931609,-0.0319781962225358,
0.076428809978167));
#62435=CARTESIAN_POINT('Ctrl Pts',(0.00794469937310318,-0.0320186447247393,
0.0765285726773943));
#62436=CARTESIAN_POINT('Ctrl Pts',(0.00894927041430031,-0.0320995417291451,
0.0763879114871669));
#62437=CARTESIAN_POINT('Ctrl Pts',(0.00943299421279664,-0.032139990231348,
0.0761469018867863));
#62438=CARTESIAN_POINT('Ctrl Pts',(0.0101564533217469,-0.0322208872357532,
0.0754029570343451));
#62439=CARTESIAN_POINT('Ctrl Pts',(0.0103931454890576,-0.0322613357379553,
0.0749015233854856));
#62440=CARTESIAN_POINT('Ctrl Pts',(0.0104828841518005,-0.0323328667545812,
0.0739661159625376));
#62441=CARTESIAN_POINT('Ctrl Pts',(0.0104111042940494,-0.0323639492690025,
0.0735454439187662));
#62442=CARTESIAN_POINT('Ctrl Pts',(0.0102368137674672,-0.0323950317834238,
0.0731679328567764));
#62443=CARTESIAN_POINT('Ctrl Pts',(0.00814801668780212,-0.0211072579114564,
0.07605678506462));
#62444=CARTESIAN_POINT('Ctrl Pts',(0.00835212411518636,-0.0211255606965017,
0.076056125656151));
#62445=CARTESIAN_POINT('Ctrl Pts',(0.00855476749622787,-0.0211438634815471,
0.0760235656396361));
#62446=CARTESIAN_POINT('Ctrl Pts',(0.00939708426598712,-0.0212246662665928,
0.0757338805617789));
#62447=CARTESIAN_POINT('Ctrl Pts',(0.00988702802146066,-0.0212871662665918,
0.0751430794075642));
#62448=CARTESIAN_POINT('Ctrl Pts',(0.0101232087195095,-0.0214121662665932,
0.0738376922384734));
#62449=CARTESIAN_POINT('Ctrl Pts',(0.00987324480820894,-0.021474666266593,
0.073147689549446));
#62450=CARTESIAN_POINT('Ctrl Pts',(0.0089167610235679,-0.0215996662665919,
0.0722962388864693));
#62451=CARTESIAN_POINT('Ctrl Pts',(0.00822945225385138,-0.0216621662665925,
0.0721430341238275));
#62452=CARTESIAN_POINT('Ctrl Pts',(0.00703231984039108,-0.0217871662665924,
0.0724624609241718));
#62453=CARTESIAN_POINT('Ctrl Pts',(0.00653742293657822,-0.0218496662665923,
0.0729254531013723));
#62454=CARTESIAN_POINT('Ctrl Pts',(0.00612213906812888,-0.0219746662665926,
0.0740526572687589));
#62455=CARTESIAN_POINT('Ctrl Pts',(0.0062024986305861,-0.0220371662665924,
0.0747016337122979));
#62456=CARTESIAN_POINT('Ctrl Pts',(0.00683777690670826,-0.0221621662665925,
0.0756803008502788));
#62457=CARTESIAN_POINT('Ctrl Pts',(0.00738258273676963,-0.0222246662665922,
0.0760014915719832));
#62458=CARTESIAN_POINT('Ctrl Pts',(0.00851285299155973,-0.0223496662665927,
0.0761060218805955));
#62459=CARTESIAN_POINT('Ctrl Pts',(0.00908700825207452,-0.0224121662665926,
0.0758916126988471));
#62460=CARTESIAN_POINT('Ctrl Pts',(0.009867934505352,-0.0225371662665923,
0.0751086198167669));
#62461=CARTESIAN_POINT('Ctrl Pts',(0.0100698264375556,-0.0225996662665926,
0.0745489205445409));
#62462=CARTESIAN_POINT('Ctrl Pts',(0.00999137500636933,-0.0227246662665924,
0.0734730045098974));
#62463=CARTESIAN_POINT('Ctrl Pts',(0.00971409165292503,-0.0227871662665921,
0.0729652157409598));
#62464=CARTESIAN_POINT('Ctrl Pts',(0.00888282738880219,-0.0229121662665928,
0.0723178841967402));
#62465=CARTESIAN_POINT('Ctrl Pts',(0.00833621828939995,-0.0229746662665921,
0.0721813898931065));
#62466=CARTESIAN_POINT('Ctrl Pts',(0.00731858981585824,-0.0230996662665929,
0.0723410721157334));
#62467=CARTESIAN_POINT('Ctrl Pts',(0.00685408613370773,-0.0231621662665927,
0.0726343422814147));
#62468=CARTESIAN_POINT('Ctrl Pts',(0.00627188449978499,-0.0232871662665922,
0.0734573086233949));
#62469=CARTESIAN_POINT('Ctrl Pts',(0.00615642736772064,-0.0233496662665926,
0.07398099780415));
#62470=CARTESIAN_POINT('Ctrl Pts',(0.00632058686144516,-0.0234746662665924,
0.0749546945714818));
#62471=CARTESIAN_POINT('Ctrl Pts',(0.00659784007307093,-0.0235371662665921,
0.0753994199917464));
#62472=CARTESIAN_POINT('Ctrl Pts',(0.007376147995406,-0.0236621662665928,
0.075974991173125));
#62473=CARTESIAN_POINT('Ctrl Pts',(0.00787234780121979,-0.0237246662665926,
0.0761038540413805));
#62474=CARTESIAN_POINT('Ctrl Pts',(0.00881571254739481,-0.0238496662665925,
0.0759944503948627));
#62475=CARTESIAN_POINT('Ctrl Pts',(0.00925841300542465,-0.0239121662665925,
0.0757578644326881));
#62476=CARTESIAN_POINT('Ctrl Pts',(0.0098711682512917,-0.0240371662665925,
0.0750551282138252));
#62477=CARTESIAN_POINT('Ctrl Pts',(0.0100392249004471,-0.0240996662665926,
0.0745928466798487));
#62478=CARTESIAN_POINT('Ctrl Pts',(0.0100319815915929,-0.0242246662665924,
0.0736769154324963));
#62479=CARTESIAN_POINT('Ctrl Pts',(0.0098576459212449,-0.0242871662665928,
0.0732271346566689));
#62480=CARTESIAN_POINT('Ctrl Pts',(0.00926368508465529,-0.0244121662665922,
0.0725504421633576));
#62481=CARTESIAN_POINT('Ctrl Pts',(0.00884704504328137,-0.0244746662665927,
0.0723256519701696));
#62482=CARTESIAN_POINT('Ctrl Pts',(0.00797138179410088,-0.0245996662665922,
0.07219343949548));
#62483=CARTESIAN_POINT('Ctrl Pts',(0.00751572112090685,-0.0246621662665923,
0.0722857508103344));
#62484=CARTESIAN_POINT('Ctrl Pts',(0.00676795485175628,-0.0247871662665926,
0.0727333505959289));
#62485=CARTESIAN_POINT('Ctrl Pts',(0.00647809666942974,-0.0248496662665925,
0.073086482268025));
#62486=CARTESIAN_POINT('Ctrl Pts',(0.00618146533527733,-0.0249746662665924,
0.0738916281021063));
#62487=CARTESIAN_POINT('Ctrl Pts',(0.00617506843092123,-0.0250371662665924,
0.0743407833313369));
#62488=CARTESIAN_POINT('Ctrl Pts',(0.00643703700353636,-0.0251621662665925,
0.0751443712971177));
#62489=CARTESIAN_POINT('Ctrl Pts',(0.00670404041284908,-0.0252246662665924,
0.0754965010570941));
#62490=CARTESIAN_POINT('Ctrl Pts',(0.00739271373153814,-0.0253496662665925,
0.0759650125972991));
#62491=CARTESIAN_POINT('Ctrl Pts',(0.00781207442037852,-0.0254121662665926,
0.0760804681250833));
#62492=CARTESIAN_POINT('Ctrl Pts',(0.00863215889728322,-0.0255371662665924,
0.0760382325197273));
#62493=CARTESIAN_POINT('Ctrl Pts',(0.0090306448835366,-0.025599666266592,
0.0758811474014697));
#62494=CARTESIAN_POINT('Ctrl Pts',(0.0096546204052879,-0.0257246662665929,
0.0753648274104897));
#62495=CARTESIAN_POINT('Ctrl Pts',(0.00987876695480732,-0.0257871662665926,
0.0750072900452153));
#62496=CARTESIAN_POINT('Ctrl Pts',(0.0100752103419703,-0.0259121662665923,
0.0742327400711651));
#62497=CARTESIAN_POINT('Ctrl Pts',(0.0100474244538565,-0.0259746662665924,
0.0738177503330937));
#62498=CARTESIAN_POINT('Ctrl Pts',(0.00975897010215047,-0.0260996662665926,
0.0730837214741746));
#62499=CARTESIAN_POINT('Ctrl Pts',(0.00949934019014137,-0.0261621662665928,
0.0727662697552228));
#62500=CARTESIAN_POINT('Ctrl Pts',(0.00884867337874248,-0.0262871662665921,
0.0723385359604954));
#62501=CARTESIAN_POINT('Ctrl Pts',(0.00845929038676506,-0.0263496662665926,
0.0722289127955772));
#62502=CARTESIAN_POINT('Ctrl Pts',(0.00769050740141413,-0.0264746662665923,
0.0722485755987396));
#62503=CARTESIAN_POINT('Ctrl Pts',(0.0073127385103659,-0.0265371662665915,
0.0723774872479133));
#62504=CARTESIAN_POINT('Ctrl Pts',(0.00669672771899448,-0.0266621662665934,
0.0728221789114253));
#62505=CARTESIAN_POINT('Ctrl Pts',(0.00645955767124918,-0.0267246662665926,
0.0731368026319471));
#62506=CARTESIAN_POINT('Ctrl Pts',(0.00611222183958379,-0.0268919420154909,
0.0740795755859367));
#62507=CARTESIAN_POINT('Ctrl Pts',(0.00620960829772417,-0.0269967177643891,
0.0747851908841829));
#62508=CARTESIAN_POINT('Ctrl Pts',(0.00698099751955323,-0.0272062692621875,
0.0758117979253375));
#62509=CARTESIAN_POINT('Ctrl Pts',(0.00764579640796796,-0.0273110450110865,
0.0761138323326925));
#62510=CARTESIAN_POINT('Ctrl Pts',(0.00895151249954563,-0.0275205965088817,
0.0759939008582095));
#62511=CARTESIAN_POINT('Ctrl Pts',(0.00956921024717631,-0.0276253722577802,
0.0755695035082156));
#62512=CARTESIAN_POINT('Ctrl Pts',(0.0101391127975682,-0.0278349237555796,
0.0743566277259409));
#62513=CARTESIAN_POINT('Ctrl Pts',(0.0100758233948543,-0.0279396995044774,
0.0735890033938645));
#62514=CARTESIAN_POINT('Ctrl Pts',(0.00927465732816471,-0.028149251002274,
0.0724764802177239));
#62515=CARTESIAN_POINT('Ctrl Pts',(0.00854863504798854,-0.0282540267511745,
0.0721581017954751));
#62516=CARTESIAN_POINT('Ctrl Pts',(0.0071586286123545,-0.0284635782489686,
0.0723565014738116));
#62517=CARTESIAN_POINT('Ctrl Pts',(0.00652722395860935,-0.0285683539978693,
0.0728754416319487));
#62518=CARTESIAN_POINT('Ctrl Pts',(0.0061941131930515,-0.0287255176212164,
0.0739025770922874));
#62519=CARTESIAN_POINT('Ctrl Pts',(0.00618172482778142,-0.0287779054956661,
0.0742791192866981));
#62520=CARTESIAN_POINT('Ctrl Pts',(0.00636558444125528,-0.0288826812445643,
0.0749848648164158));
#62521=CARTESIAN_POINT('Ctrl Pts',(0.00656179628659944,-0.0289350691190143,
0.0753127819778567));
#62522=CARTESIAN_POINT('Ctrl Pts',(0.0071076452778826,-0.0290398448679119,
0.0758111224113399));
#62523=CARTESIAN_POINT('Ctrl Pts',(0.00745650463288417,-0.0290922327423619,
0.0759804115890255));
#62524=CARTESIAN_POINT('Ctrl Pts',(0.00819673799450679,-0.0291970084912602,
0.0760968804211664));
#62525=CARTESIAN_POINT('Ctrl Pts',(0.00858674947338286,-0.0292493963657099,
0.0760435018440831));
#62526=CARTESIAN_POINT('Ctrl Pts',(0.00927564963473071,-0.0293541721146081,
0.0757225423137761));
#62527=CARTESIAN_POINT('Ctrl Pts',(0.00957299018710003,-0.029406559989058,
0.0754552752219081));
#62528=CARTESIAN_POINT('Ctrl Pts',(0.00996560701721403,-0.0295113357379557,
0.0747915828297948));
#62529=CARTESIAN_POINT('Ctrl Pts',(0.010059696968687,-0.0295637236124048,
0.074396372440036));
#62530=CARTESIAN_POINT('Ctrl Pts',(0.0100007835149004,-0.0296684993613048,
0.0736158357642392));
#62531=CARTESIAN_POINT('Ctrl Pts',(0.00984747524688978,-0.0297208872357529,
0.073232313186738));
#62532=CARTESIAN_POINT('Ctrl Pts',(0.00933890234319653,-0.0298256629846524,
0.0726213568608565));
#62533=CARTESIAN_POINT('Ctrl Pts',(0.00898449292909369,-0.0298780508591023,
0.0723957035479018));
#62534=CARTESIAN_POINT('Ctrl Pts',(0.00820150519090858,-0.0299828266079989,
0.0721974790286785));
#62535=CARTESIAN_POINT('Ctrl Pts',(0.00777480494848981,-0.03003521448245,
0.072225929314564));
#62536=CARTESIAN_POINT('Ctrl Pts',(0.00701567178618897,-0.030139990231347,
0.0725388127232768));
#62537=CARTESIAN_POINT('Ctrl Pts',(0.00668553723143537,-0.030192378105796,
0.0728229295147053));
#62538=CARTESIAN_POINT('Ctrl Pts',(0.00626320349708927,-0.0302971538546968,
0.0735434428689412));
#62539=CARTESIAN_POINT('Ctrl Pts',(0.00617279507523841,-0.0303495417291453,
0.0739780598173242));
#62540=CARTESIAN_POINT('Ctrl Pts',(0.00628368831566111,-0.0304543174780433,
0.0748207970461326));
#62541=CARTESIAN_POINT('Ctrl Pts',(0.00648535233659179,-0.0305067053524937,
0.0752261858068767));
#62542=CARTESIAN_POINT('Ctrl Pts',(0.00710862553564354,-0.0306114811013907,
0.0758269273212183));
#62543=CARTESIAN_POINT('Ctrl Pts',(0.00752869276012381,-0.03066386897584,
0.0760196869779353));
#62544=CARTESIAN_POINT('Ctrl Pts',(0.00840797945427604,-0.0307686447247403,
0.076091415138353));
#62545=CARTESIAN_POINT('Ctrl Pts',(0.00886408949546226,-0.0308210325991885,
0.075969235922541));
#62546=CARTESIAN_POINT('Ctrl Pts',(0.00959764252618967,-0.0309258083480876,
0.0754482333981525));
#62547=CARTESIAN_POINT('Ctrl Pts',(0.00987164018299474,-0.0309781962225361,
0.0750506297150497));
#62548=CARTESIAN_POINT('Ctrl Pts',(0.0100900140080253,-0.0310829719714357,
0.07415859534242));
#62549=CARTESIAN_POINT('Ctrl Pts',(0.0100323696451357,-0.031135359845885,
0.0736676702543576));
#62550=CARTESIAN_POINT('Ctrl Pts',(0.00959236173346572,-0.0312401355947827,
0.0728390376922328));
#62551=CARTESIAN_POINT('Ctrl Pts',(0.00921089015096985,-0.0312925234692314,
0.0725057397900231));
#62552=CARTESIAN_POINT('Ctrl Pts',(0.00830589411414326,-0.0313972992181321,
0.0721872899879916));
#62553=CARTESIAN_POINT('Ctrl Pts',(0.00778642158836204,-0.0314496870925817,
0.0722051113571944));
#62554=CARTESIAN_POINT('Ctrl Pts',(0.00689097003953919,-0.0315544628414776,
0.0726083845495457));
#62555=CARTESIAN_POINT('Ctrl Pts',(0.00652059245595663,-0.0316068507159279,
0.0729931501375565));
#62556=CARTESIAN_POINT('Ctrl Pts',(0.00615880568740368,-0.0317116264648272,
0.0739323161427358));
#62557=CARTESIAN_POINT('Ctrl Pts',(0.00617138346343902,-0.031764014339277,
0.0744817452447779));
#62558=CARTESIAN_POINT('Ctrl Pts',(0.00655457842863585,-0.0318568507159276,
0.0753126836656081));
#62559=CARTESIAN_POINT('Ctrl Pts',(0.00684017822748756,-0.0318972992181318,
0.0756242331860024));
#62560=CARTESIAN_POINT('Ctrl Pts',(0.00755208080592647,-0.0319781962225358,
0.0760192672747625));
#62561=CARTESIAN_POINT('Ctrl Pts',(0.0079768837425508,-0.0320186447247393,
0.0761011008417093));
#62562=CARTESIAN_POINT('Ctrl Pts',(0.00880091549178614,-0.0320995417291451,
0.0759857189703642));
#62563=CARTESIAN_POINT('Ctrl Pts',(0.00919770551606028,-0.032139990231348,
0.0757880230838218));
#62564=CARTESIAN_POINT('Ctrl Pts',(0.00979114614952519,-0.0322208872357532,
0.0751777783595053));
#62565=CARTESIAN_POINT('Ctrl Pts',(0.00998530052254685,-0.0322613357379553,
0.0747664612601165));
#62566=CARTESIAN_POINT('Ctrl Pts',(0.0100589115507385,-0.0323328667545812,
0.0739991631961976));
#62567=CARTESIAN_POINT('Ctrl Pts',(0.0100000318107133,-0.0323639492690025,
0.0736540934043486));
#62568=CARTESIAN_POINT('Ctrl Pts',(0.00985706439317406,-0.0323950317834238,
0.0733444277978263));
#62569=CARTESIAN_POINT('Ctrl Pts',(0.0081456011935425,-0.0209166974216957,
0.0758667324789935));
#62570=CARTESIAN_POINT('Ctrl Pts',(0.00832936487844643,-0.020935000206741,
0.0758661387949141));
#62571=CARTESIAN_POINT('Ctrl Pts',(0.00851181044105437,-0.0209533029917864,
0.075836824091907));
#62572=CARTESIAN_POINT('Ctrl Pts',(0.00927017203255066,-0.0210341057768321,
0.075576012429877));
#62573=CARTESIAN_POINT('Ctrl Pts',(0.0097112822413036,-0.0210966057768311,
0.0750440974548303));
#62574=CARTESIAN_POINT('Ctrl Pts',(0.00992392239817022,-0.0212216057768325,
0.0738688204965506));
#62575=CARTESIAN_POINT('Ctrl Pts',(0.00969887282490249,-0.0212841057768323,
0.0732475915762989));
#62576=CARTESIAN_POINT('Ctrl Pts',(0.00883772344357415,-0.0214091057768312,
0.0724810064826171));
#62577=CARTESIAN_POINT('Ctrl Pts',(0.00821891993500742,-0.0214716057768319,
0.0723430719052785));
#62578=CARTESIAN_POINT('Ctrl Pts',(0.00714110779247693,-0.0215966057768317,
0.072630660880558));
#62579=CARTESIAN_POINT('Ctrl Pts',(0.00669553812429927,-0.0216591057768317,
0.0730475058217461));
#62580=CARTESIAN_POINT('Ctrl Pts',(0.00632164632170585,-0.0217841057768319,
0.07406235958818));
#62581=CARTESIAN_POINT('Ctrl Pts',(0.00639399630672924,-0.0218466057768317,
0.0746466514202262));
#62582=CARTESIAN_POINT('Ctrl Pts',(0.00696595529154281,-0.0219716057768319,
0.075527773101463));
#62583=CARTESIAN_POINT('Ctrl Pts',(0.00745645937643706,-0.0220341057768316,
0.0758169501849909));
#62584=CARTESIAN_POINT('Ctrl Pts',(0.00847407362800718,-0.0221591057768321,
0.0759110617758377));
#62585=CARTESIAN_POINT('Ctrl Pts',(0.00899100183454682,-0.0222216057768319,
0.0757180231303543));
#62586=CARTESIAN_POINT('Ctrl Pts',(0.00969409180917257,-0.0223466057768317,
0.0750130725114152));
#62587=CARTESIAN_POINT('Ctrl Pts',(0.00987586082115598,-0.0224091057768319,
0.0745091594396549));
#62588=CARTESIAN_POINT('Ctrl Pts',(0.00980522878063905,-0.0225341057768317,
0.0735404818285206));
#62589=CARTESIAN_POINT('Ctrl Pts',(0.00955558274156816,-0.0225966057768315,
0.07308330524985));
#62590=CARTESIAN_POINT('Ctrl Pts',(0.00880717203323765,-0.0227216057768321,
0.0725004943671456));
#62591=CARTESIAN_POINT('Ctrl Pts',(0.00831504441399582,-0.0227841057768314,
0.072377604688286));
#62592=CARTESIAN_POINT('Ctrl Pts',(0.00739884474131507,-0.0229091057768322,
0.0725213711059004));
#62593=CARTESIAN_POINT('Ctrl Pts',(0.00698063894950555,-0.0229716057768321,
0.0727854105238122));
#62594=CARTESIAN_POINT('Ctrl Pts',(0.00645646636559797,-0.0230966057768316,
0.0735263503783403));
#62595=CARTESIAN_POINT('Ctrl Pts',(0.00635251704680801,-0.023159105776832,
0.0739978425471124));
#62596=CARTESIAN_POINT('Ctrl Pts',(0.00650031447811829,-0.0232841057768316,
0.0748744892631922));
#62597=CARTESIAN_POINT('Ctrl Pts',(0.00674993337965833,-0.0233466057768315,
0.0752748881268966));
#62598=CARTESIAN_POINT('Ctrl Pts',(0.00745066599694304,-0.0234716057768321,
0.0757930911270036));
#62599=CARTESIAN_POINT('Ctrl Pts',(0.00789740870461186,-0.0235341057768318,
0.0759091100089296));
#62600=CARTESIAN_POINT('Ctrl Pts',(0.00874674664486829,-0.0236591057768317,
0.0758106108142473));
#62601=CARTESIAN_POINT('Ctrl Pts',(0.00914532237784772,-0.0237216057768318,
0.0755976057866355));
#62602=CARTESIAN_POINT('Ctrl Pts',(0.00969700324202693,-0.0238466057768318,
0.0749649125096261));
#62603=CARTESIAN_POINT('Ctrl Pts',(0.00984830939250459,-0.0239091057768318,
0.0745487073806151));
#62604=CARTESIAN_POINT('Ctrl Pts',(0.00984178803684884,-0.0240341057768317,
0.0737240685946132));
#62605=CARTESIAN_POINT('Ctrl Pts',(0.00968482870614778,-0.0240966057768321,
0.0733191182514325));
#62606=CARTESIAN_POINT('Ctrl Pts',(0.00915006897976686,-0.0242216057768316,
0.0727098728765269));
#62607=CARTESIAN_POINT('Ctrl Pts',(0.00877495617636422,-0.0242841057768321,
0.0725074879130797));
#62608=CARTESIAN_POINT('Ctrl Pts',(0.00798657180708102,-0.0244091057768316,
0.0723884532858218));
#62609=CARTESIAN_POINT('Ctrl Pts',(0.00757632762613652,-0.0244716057768317,
0.0724715637712821));
#62610=CARTESIAN_POINT('Ctrl Pts',(0.00690309252231404,-0.0245966057768319,
0.072874550507322));
#62611=CARTESIAN_POINT('Ctrl Pts',(0.00664212500943859,-0.0246591057768318,
0.0731924849311315));
#62612=CARTESIAN_POINT('Ctrl Pts',(0.0063750594365665,-0.0247841057768317,
0.0739173804787947));
#62613=CARTESIAN_POINT('Ctrl Pts',(0.00636930012279967,-0.0248466057768317,
0.0743217676246966));
#62614=CARTESIAN_POINT('Ctrl Pts',(0.00660515783189783,-0.0249716057768318,
0.0750452605795038));
#62615=CARTESIAN_POINT('Ctrl Pts',(0.00684554854675824,-0.0250341057768317,
0.0753622929535182));
#62616=CARTESIAN_POINT('Ctrl Pts',(0.00746558059732679,-0.0251591057768318,
0.0757841071331952));
#62617=CARTESIAN_POINT('Ctrl Pts',(0.00784314287652831,-0.0252216057768319,
0.0758880550076066));
#62618=CARTESIAN_POINT('Ctrl Pts',(0.00858148810648805,-0.0253466057768317,
0.0758500290985359));
#62619=CARTESIAN_POINT('Ctrl Pts',(0.00894025630103604,-0.0254091057768313,
0.0757086009273785));
#62620=CARTESIAN_POINT('Ctrl Pts',(0.00950203909667648,-0.0255341057768323,
0.0752437434484126));
#62621=CARTESIAN_POINT('Ctrl Pts',(0.00970384456953965,-0.025596605776832,
0.0749218424545307));
#62622=CARTESIAN_POINT('Ctrl Pts',(0.00988070810244839,-0.0257216057768316,
0.0742244932242857));
#62623=CARTESIAN_POINT('Ctrl Pts',(0.00985569168215658,-0.0257841057768317,
0.0738508662355836));
#62624=CARTESIAN_POINT('Ctrl Pts',(0.0095959880776607,-0.0259091057768319,
0.0731899993104086));
#62625=CARTESIAN_POINT('Ctrl Pts',(0.0093622359307961,-0.0259716057768321,
0.0729041885567222));
#62626=CARTESIAN_POINT('Ctrl Pts',(0.00877642221279626,-0.0260966057768315,
0.0725190877336685));
#62627=CARTESIAN_POINT('Ctrl Pts',(0.00842584970124339,-0.0261591057768319,
0.0724203909003668));
#62628=CARTESIAN_POINT('Ctrl Pts',(0.00773369265389813,-0.0262841057768317,
0.0724380938777203));
#62629=CARTESIAN_POINT('Ctrl Pts',(0.00739357664562364,-0.0263466057768309,
0.0725541566784855));
#62630=CARTESIAN_POINT('Ctrl Pts',(0.00683896472182591,-0.0264716057768327,
0.0729545251500316));
#62631=CARTESIAN_POINT('Ctrl Pts',(0.0066254338254687,-0.0265341057768319,
0.0732377897768127));
#62632=CARTESIAN_POINT('Ctrl Pts',(0.00631271756058805,-0.0267013815257303,
0.0740865949098408));
#62633=CARTESIAN_POINT('Ctrl Pts',(0.00640039734097116,-0.0268061572746284,
0.0747218803033809));
#62634=CARTESIAN_POINT('Ctrl Pts',(0.00709490085666943,-0.0270157087724267,
0.0756461636342162));
#62635=CARTESIAN_POINT('Ctrl Pts',(0.00769343808297591,-0.0271204845213259,
0.0759180937465821));
#62636=CARTESIAN_POINT('Ctrl Pts',(0.00886901117946571,-0.027330036019121,
0.0758101160508686));
#62637=CARTESIAN_POINT('Ctrl Pts',(0.00942514191765672,-0.0274348117680204,
0.0754280191232956));
#62638=CARTESIAN_POINT('Ctrl Pts',(0.00993824128909218,-0.027644363265818,
0.0743360327809175));
#62639=CARTESIAN_POINT('Ctrl Pts',(0.00988126005128462,-0.0277491390147176,
0.0736449189018586));
#62640=CARTESIAN_POINT('Ctrl Pts',(0.00915994760067147,-0.0279586905125125,
0.072643282846725));
#62641=CARTESIAN_POINT('Ctrl Pts',(0.00850628922460295,-0.028063466261413,
0.0723566377558719));
#62642=CARTESIAN_POINT('Ctrl Pts',(0.00725482714933299,-0.0282730177592087,
0.0725352625930086));
#62643=CARTESIAN_POINT('Ctrl Pts',(0.00668635569621314,-0.0283777935081086,
0.0730024790825113));
#62644=CARTESIAN_POINT('Ctrl Pts',(0.00638644666034619,-0.0285349571314557,
0.0739272381640707));
#62645=CARTESIAN_POINT('Ctrl Pts',(0.00637529306500116,-0.0285873450059055,
0.0742662497426962));
#62646=CARTESIAN_POINT('Ctrl Pts',(0.00654082707084289,-0.0286921207548037,
0.0749016523873107));
#62647=CARTESIAN_POINT('Ctrl Pts',(0.00671748214010876,-0.0287445086292537,
0.0751968854746209));
#62648=CARTESIAN_POINT('Ctrl Pts',(0.00720892541253046,-0.0288492843781513,
0.0756455554498743));
#62649=CARTESIAN_POINT('Ctrl Pts',(0.00752301334852511,-0.0289016722526012,
0.0757979712806186));
#62650=CARTESIAN_POINT('Ctrl Pts',(0.00818946636282185,-0.0290064480014996,
0.0759028314615779));
#62651=CARTESIAN_POINT('Ctrl Pts',(0.00854060471889044,-0.0290588358759492,
0.0758547732201633));
#62652=CARTESIAN_POINT('Ctrl Pts',(0.00916084100231525,-0.0291636116248473,
0.075565804284784));
#62653=CARTESIAN_POINT('Ctrl Pts',(0.00942854510439027,-0.0292159994992974,
0.0753251761690674));
#62654=CARTESIAN_POINT('Ctrl Pts',(0.00978202913180507,-0.029320775248195,
0.0747276351526504));
#62655=CARTESIAN_POINT('Ctrl Pts',(0.00986674097407697,-0.029373163122644,
0.074371816070194));
#62656=CARTESIAN_POINT('Ctrl Pts',(0.00981369952675195,-0.0294779388715441,
0.0736690768431837));
#62657=CARTESIAN_POINT('Ctrl Pts',(0.00967567176060491,-0.0295303267459923,
0.0733237806283977));
#62658=CARTESIAN_POINT('Ctrl Pts',(0.00921778920325428,-0.0296351024948917,
0.0727737193827185));
#62659=CARTESIAN_POINT('Ctrl Pts',(0.00889870439220733,-0.0296874903693416,
0.0725705573281537));
#62660=CARTESIAN_POINT('Ctrl Pts',(0.00819375840446231,-0.0297922661182383,
0.0723920901917167));
#62661=CARTESIAN_POINT('Ctrl Pts',(0.00780958811776,-0.0298446539926894,
0.0724177047880981));
#62662=CARTESIAN_POINT('Ctrl Pts',(0.00712611907880853,-0.0299494297415862,
0.0726994025629769));
#62663=CARTESIAN_POINT('Ctrl Pts',(0.00682888960963579,-0.0300018176160353,
0.0729552009393765));
#62664=CARTESIAN_POINT('Ctrl Pts',(0.0064486506135478,-0.0301065933649361,
0.07360389947374));
#62665=CARTESIAN_POINT('Ctrl Pts',(0.00636725335643387,-0.0301589812393846,
0.0739951973945462));
#62666=CARTESIAN_POINT('Ctrl Pts',(0.00646709367460444,-0.0302637569882826,
0.0747539375372065));
#62667=CARTESIAN_POINT('Ctrl Pts',(0.00664865749162809,-0.0303161448627331,
0.0751189204946994));
#62668=CARTESIAN_POINT('Ctrl Pts',(0.00720980796629447,-0.03042092061163,
0.0756597850568809));
#62669=CARTESIAN_POINT('Ctrl Pts',(0.00758800635949914,-0.0304733084860793,
0.0758333320231676));
#62670=CARTESIAN_POINT('Ctrl Pts',(0.00837965301868817,-0.0305780842349796,
0.0758979109130133));
#62671=CARTESIAN_POINT('Ctrl Pts',(0.0087903017783351,-0.0306304721094278,
0.0757879095122608));
#62672=CARTESIAN_POINT('Ctrl Pts',(0.00945074030194221,-0.030735247858327,
0.0753188362161399));
#62673=CARTESIAN_POINT('Ctrl Pts',(0.00969742813547587,-0.0307876357327754,
0.074960862384052));
#62674=CARTESIAN_POINT('Ctrl Pts',(0.00989403626134592,-0.030892411481675,
0.0741577386296832));
#62675=CARTESIAN_POINT('Ctrl Pts',(0.00984213741241968,-0.0309447993561243,
0.0737157448994683));
#62676=CARTESIAN_POINT('Ctrl Pts',(0.00944598585501893,-0.031049575105022,
0.0729697035868178));
#62677=CARTESIAN_POINT('Ctrl Pts',(0.0091025362089969,-0.0311019629794706,
0.0726696260665349));
#62678=CARTESIAN_POINT('Ctrl Pts',(0.00828774270205792,-0.0312067387283715,
0.0723829167104463));
#62679=CARTESIAN_POINT('Ctrl Pts',(0.00782004690692066,-0.031259126602821,
0.0723989617927675));
#62680=CARTESIAN_POINT('Ctrl Pts',(0.00701384657225643,-0.0313639023517169,
0.0727620400442508));
#62681=CARTESIAN_POINT('Ctrl Pts',(0.00668038516697007,-0.0314162902261672,
0.0731084553765258));
#62682=CARTESIAN_POINT('Ctrl Pts',(0.00635465831522934,-0.0315210659750665,
0.0739540130716083));
#62683=CARTESIAN_POINT('Ctrl Pts',(0.00636598244243914,-0.0315734538495163,
0.0744486796189194));
#62684=CARTESIAN_POINT('Ctrl Pts',(0.00671098369860905,-0.0316662902261669,
0.0751967969613253));
#62685=CARTESIAN_POINT('Ctrl Pts',(0.00696811726850124,-0.0317067387283712,
0.0754772937988554));
#62686=CARTESIAN_POINT('Ctrl Pts',(0.00760906327807618,-0.0317876357327751,
0.0758329541525405));
#62687=CARTESIAN_POINT('Ctrl Pts',(0.00799152536675427,-0.0318280842349786,
0.0759066312254608));
#62688=CARTESIAN_POINT('Ctrl Pts',(0.00873342443754237,-0.0319089812393844,
0.0758027496660232));
#62689=CARTESIAN_POINT('Ctrl Pts',(0.00909066570959304,-0.0319494297415873,
0.0756247584725279));
#62690=CARTESIAN_POINT('Ctrl Pts',(0.00962495708239995,-0.0320303267459926,
0.0750753379018474));
#62691=CARTESIAN_POINT('Ctrl Pts',(0.00979975975119023,-0.0320707752481946,
0.0747050174935392));
#62692=CARTESIAN_POINT('Ctrl Pts',(0.00986603384010217,-0.0321423062648206,
0.0740141973629227));
#62693=CARTESIAN_POINT('Ctrl Pts',(0.00981302274622929,-0.0321733887792418,
0.0737035212777265));
#62694=CARTESIAN_POINT('Ctrl Pts',(0.00968430513999177,-0.0322044712936632,
0.0734247205810942));
#62695=CARTESIAN_POINT('Ctrl Pts',(0.0081456011935425,-0.0204978184012171,
0.0758667324789935));
#62696=CARTESIAN_POINT('Ctrl Pts',(0.00832936487844643,-0.0205161211862624,
0.0758661387949141));
#62697=CARTESIAN_POINT('Ctrl Pts',(0.00851181044105437,-0.0205344239713078,
0.075836824091907));
#62698=CARTESIAN_POINT('Ctrl Pts',(0.00927017203255066,-0.0206152267563535,
0.075576012429877));
#62699=CARTESIAN_POINT('Ctrl Pts',(0.0097112822413036,-0.0206777267563525,
0.0750440974548303));
#62700=CARTESIAN_POINT('Ctrl Pts',(0.00992392239817022,-0.0208027267563538,
0.0738688204965506));
#62701=CARTESIAN_POINT('Ctrl Pts',(0.00969887282490249,-0.0208652267563538,
0.0732475915762989));
#62702=CARTESIAN_POINT('Ctrl Pts',(0.00883772344357415,-0.0209902267563526,
0.0724810064826171));
#62703=CARTESIAN_POINT('Ctrl Pts',(0.00821891993500742,-0.0210527267563532,
0.0723430719052785));
#62704=CARTESIAN_POINT('Ctrl Pts',(0.00714110779247693,-0.0211777267563531,
0.072630660880558));
#62705=CARTESIAN_POINT('Ctrl Pts',(0.00669553812429927,-0.0212402267563531,
0.0730475058217461));
#62706=CARTESIAN_POINT('Ctrl Pts',(0.00632164632170585,-0.0213652267563533,
0.07406235958818));
#62707=CARTESIAN_POINT('Ctrl Pts',(0.00639399630672924,-0.0214277267563531,
0.0746466514202262));
#62708=CARTESIAN_POINT('Ctrl Pts',(0.00696595529154281,-0.0215527267563532,
0.075527773101463));
#62709=CARTESIAN_POINT('Ctrl Pts',(0.00745645937643706,-0.0216152267563529,
0.0758169501849909));
#62710=CARTESIAN_POINT('Ctrl Pts',(0.00847407362800718,-0.0217402267563534,
0.0759110617758377));
#62711=CARTESIAN_POINT('Ctrl Pts',(0.00899100183454682,-0.0218027267563532,
0.0757180231303543));
#62712=CARTESIAN_POINT('Ctrl Pts',(0.00969409180917257,-0.0219277267563531,
0.0750130725114152));
#62713=CARTESIAN_POINT('Ctrl Pts',(0.00987586082115598,-0.0219902267563532,
0.0745091594396549));
#62714=CARTESIAN_POINT('Ctrl Pts',(0.00980522878063905,-0.0221152267563531,
0.0735404818285206));
#62715=CARTESIAN_POINT('Ctrl Pts',(0.00955558274156816,-0.0221777267563529,
0.07308330524985));
#62716=CARTESIAN_POINT('Ctrl Pts',(0.00880717203323765,-0.0223027267563535,
0.0725004943671456));
#62717=CARTESIAN_POINT('Ctrl Pts',(0.00831504441399582,-0.0223652267563527,
0.072377604688286));
#62718=CARTESIAN_POINT('Ctrl Pts',(0.00739884474131507,-0.0224902267563536,
0.0725213711059004));
#62719=CARTESIAN_POINT('Ctrl Pts',(0.00698063894950555,-0.0225527267563534,
0.0727854105238122));
#62720=CARTESIAN_POINT('Ctrl Pts',(0.00645646636559797,-0.0226777267563529,
0.0735263503783403));
#62721=CARTESIAN_POINT('Ctrl Pts',(0.00635251704680801,-0.0227402267563533,
0.0739978425471124));
#62722=CARTESIAN_POINT('Ctrl Pts',(0.00650031447811829,-0.022865226756353,
0.0748744892631922));
#62723=CARTESIAN_POINT('Ctrl Pts',(0.00674993337965833,-0.0229277267563529,
0.0752748881268966));
#62724=CARTESIAN_POINT('Ctrl Pts',(0.00745066599694304,-0.0230527267563535,
0.0757930911270036));
#62725=CARTESIAN_POINT('Ctrl Pts',(0.00789740870461186,-0.0231152267563532,
0.0759091100089296));
#62726=CARTESIAN_POINT('Ctrl Pts',(0.00874674664486829,-0.0232402267563531,
0.0758106108142473));
#62727=CARTESIAN_POINT('Ctrl Pts',(0.00914532237784772,-0.0233027267563532,
0.0755976057866355));
#62728=CARTESIAN_POINT('Ctrl Pts',(0.00969700324202693,-0.0234277267563531,
0.0749649125096261));
#62729=CARTESIAN_POINT('Ctrl Pts',(0.00984830939250459,-0.0234902267563532,
0.0745487073806151));
#62730=CARTESIAN_POINT('Ctrl Pts',(0.00984178803684884,-0.0236152267563531,
0.0737240685946132));
#62731=CARTESIAN_POINT('Ctrl Pts',(0.00968482870614778,-0.0236777267563534,
0.0733191182514325));
#62732=CARTESIAN_POINT('Ctrl Pts',(0.00915006897976686,-0.0238027267563529,
0.0727098728765269));
#62733=CARTESIAN_POINT('Ctrl Pts',(0.00877495617636422,-0.0238652267563534,
0.0725074879130797));
#62734=CARTESIAN_POINT('Ctrl Pts',(0.00798657180708102,-0.0239902267563529,
0.0723884532858218));
#62735=CARTESIAN_POINT('Ctrl Pts',(0.00757632762613652,-0.024052726756353,
0.0724715637712821));
#62736=CARTESIAN_POINT('Ctrl Pts',(0.00690309252231404,-0.0241777267563532,
0.072874550507322));
#62737=CARTESIAN_POINT('Ctrl Pts',(0.00664212500943859,-0.0242402267563532,
0.0731924849311315));
#62738=CARTESIAN_POINT('Ctrl Pts',(0.0063750594365665,-0.0243652267563532,
0.0739173804787947));
#62739=CARTESIAN_POINT('Ctrl Pts',(0.00636930012279967,-0.0244277267563531,
0.0743217676246966));
#62740=CARTESIAN_POINT('Ctrl Pts',(0.00660515783189783,-0.0245527267563532,
0.0750452605795038));
#62741=CARTESIAN_POINT('Ctrl Pts',(0.00684554854675824,-0.0246152267563531,
0.0753622929535182));
#62742=CARTESIAN_POINT('Ctrl Pts',(0.00746558059732679,-0.0247402267563532,
0.0757841071331952));
#62743=CARTESIAN_POINT('Ctrl Pts',(0.00784314287652831,-0.0248027267563532,
0.0758880550076066));
#62744=CARTESIAN_POINT('Ctrl Pts',(0.00858148810648805,-0.0249277267563531,
0.0758500290985359));
#62745=CARTESIAN_POINT('Ctrl Pts',(0.00894025630103604,-0.0249902267563527,
0.0757086009273785));
#62746=CARTESIAN_POINT('Ctrl Pts',(0.00950203909667648,-0.0251152267563537,
0.0752437434484126));
#62747=CARTESIAN_POINT('Ctrl Pts',(0.00970384456953965,-0.0251777267563533,
0.0749218424545307));
#62748=CARTESIAN_POINT('Ctrl Pts',(0.00988070810244839,-0.025302726756353,
0.0742244932242857));
#62749=CARTESIAN_POINT('Ctrl Pts',(0.00985569168215658,-0.0253652267563531,
0.0738508662355836));
#62750=CARTESIAN_POINT('Ctrl Pts',(0.0095959880776607,-0.0254902267563532,
0.0731899993104086));
#62751=CARTESIAN_POINT('Ctrl Pts',(0.00936223593079611,-0.0255527267563535,
0.0729041885567222));
#62752=CARTESIAN_POINT('Ctrl Pts',(0.00877642221279626,-0.0256777267563528,
0.0725190877336685));
#62753=CARTESIAN_POINT('Ctrl Pts',(0.00842584970124339,-0.0257402267563532,
0.0724203909003668));
#62754=CARTESIAN_POINT('Ctrl Pts',(0.00773369265389813,-0.0258652267563531,
0.0724380938777203));
#62755=CARTESIAN_POINT('Ctrl Pts',(0.00739357664562364,-0.0259277267563522,
0.0725541566784855));
#62756=CARTESIAN_POINT('Ctrl Pts',(0.00683896472182591,-0.0260527267563541,
0.0729545251500316));
#62757=CARTESIAN_POINT('Ctrl Pts',(0.0066254338254687,-0.0261152267563532,
0.0732377897768127));
#62758=CARTESIAN_POINT('Ctrl Pts',(0.00631271756058805,-0.0262825025052516,
0.0740865949098408));
#62759=CARTESIAN_POINT('Ctrl Pts',(0.00640039734097116,-0.0263872782541498,
0.0747218803033809));
#62760=CARTESIAN_POINT('Ctrl Pts',(0.00709490085666943,-0.0265968297519482,
0.0756461636342162));
#62761=CARTESIAN_POINT('Ctrl Pts',(0.00769343808297591,-0.0267016055008472,
0.0759180937465821));
#62762=CARTESIAN_POINT('Ctrl Pts',(0.00886901117946571,-0.0269111569986424,
0.0758101160508686));
#62763=CARTESIAN_POINT('Ctrl Pts',(0.00942514191765672,-0.0270159327475413,
0.0754280191232956));
#62764=CARTESIAN_POINT('Ctrl Pts',(0.00993824128909218,-0.0272254842453399,
0.0743360327809175));
#62765=CARTESIAN_POINT('Ctrl Pts',(0.00988126005128462,-0.027330259994239,
0.0736449189018586));
#62766=CARTESIAN_POINT('Ctrl Pts',(0.00915994760067147,-0.0275398114920338,
0.072643282846725));
#62767=CARTESIAN_POINT('Ctrl Pts',(0.00850628922460295,-0.0276445872409343,
0.0723566377558719));
#62768=CARTESIAN_POINT('Ctrl Pts',(0.00725482714933299,-0.0278541387387302,
0.0725352625930086));
#62769=CARTESIAN_POINT('Ctrl Pts',(0.00668635569621314,-0.0279589144876299,
0.0730024790825113));
#62770=CARTESIAN_POINT('Ctrl Pts',(0.00638644666034619,-0.028116078110977,
0.0739272381640707));
#62771=CARTESIAN_POINT('Ctrl Pts',(0.00637529306500116,-0.0281684659854268,
0.0742662497426962));
#62772=CARTESIAN_POINT('Ctrl Pts',(0.00654082707084289,-0.028273241734325,
0.0749016523873107));
#62773=CARTESIAN_POINT('Ctrl Pts',(0.00671748214010876,-0.028325629608775,
0.0751968854746209));
#62774=CARTESIAN_POINT('Ctrl Pts',(0.00720892541253046,-0.0284304053576727,
0.0756455554498743));
#62775=CARTESIAN_POINT('Ctrl Pts',(0.00752301334852511,-0.0284827932321226,
0.0757979712806186));
#62776=CARTESIAN_POINT('Ctrl Pts',(0.00818946636282185,-0.0285875689810209,
0.0759028314615779));
#62777=CARTESIAN_POINT('Ctrl Pts',(0.00854060471889044,-0.0286399568554705,
0.0758547732201633));
#62778=CARTESIAN_POINT('Ctrl Pts',(0.00916084100231525,-0.0287447326043687,
0.075565804284784));
#62779=CARTESIAN_POINT('Ctrl Pts',(0.00942854510439027,-0.0287971204788187,
0.0753251761690674));
#62780=CARTESIAN_POINT('Ctrl Pts',(0.00978202913180507,-0.0289018962277164,
0.0747276351526504));
#62781=CARTESIAN_POINT('Ctrl Pts',(0.00986674097407697,-0.0289542841021654,
0.074371816070194));
#62782=CARTESIAN_POINT('Ctrl Pts',(0.00981369952675195,-0.0290590598510655,
0.0736690768431837));
#62783=CARTESIAN_POINT('Ctrl Pts',(0.00967567176060491,-0.0291114477255137,
0.0733237806283977));
#62784=CARTESIAN_POINT('Ctrl Pts',(0.00921778920325428,-0.0292162234744131,
0.0727737193827185));
#62785=CARTESIAN_POINT('Ctrl Pts',(0.00889870439220733,-0.0292686113488629,
0.0725705573281537));
#62786=CARTESIAN_POINT('Ctrl Pts',(0.00819375840446231,-0.0293733870977596,
0.0723920901917167));
#62787=CARTESIAN_POINT('Ctrl Pts',(0.00780958811776,-0.0294257749722108,
0.0724177047880981));
#62788=CARTESIAN_POINT('Ctrl Pts',(0.00712611907880853,-0.0295305507211076,
0.0726994025629769));
#62789=CARTESIAN_POINT('Ctrl Pts',(0.00682888960963579,-0.0295829385955566,
0.0729552009393765));
#62790=CARTESIAN_POINT('Ctrl Pts',(0.0064486506135478,-0.0296877143444575,
0.07360389947374));
#62791=CARTESIAN_POINT('Ctrl Pts',(0.00636725335643387,-0.0297401022189059,
0.0739951973945462));
#62792=CARTESIAN_POINT('Ctrl Pts',(0.00646709367460444,-0.029844877967804,
0.0747539375372065));
#62793=CARTESIAN_POINT('Ctrl Pts',(0.00664865749162809,-0.0298972658422544,
0.0751189204946994));
#62794=CARTESIAN_POINT('Ctrl Pts',(0.00720980796629447,-0.0300020415911513,
0.0756597850568809));
#62795=CARTESIAN_POINT('Ctrl Pts',(0.00758800635949914,-0.0300544294656007,
0.0758333320231676));
#62796=CARTESIAN_POINT('Ctrl Pts',(0.00837965301868817,-0.0301592052145009,
0.0758979109130133));
#62797=CARTESIAN_POINT('Ctrl Pts',(0.0087903017783351,-0.0302115930889491,
0.0757879095122608));
#62798=CARTESIAN_POINT('Ctrl Pts',(0.00945074030194221,-0.0303163688378483,
0.0753188362161399));
#62799=CARTESIAN_POINT('Ctrl Pts',(0.00969742813547587,-0.0303687567122968,
0.074960862384052));
#62800=CARTESIAN_POINT('Ctrl Pts',(0.00989403626134592,-0.0304735324611964,
0.0741577386296832));
#62801=CARTESIAN_POINT('Ctrl Pts',(0.00984213741241968,-0.0305259203356456,
0.0737157448994683));
#62802=CARTESIAN_POINT('Ctrl Pts',(0.00944598585501893,-0.0306306960845434,
0.0729697035868178));
#62803=CARTESIAN_POINT('Ctrl Pts',(0.0091025362089969,-0.0306830839589921,
0.0726696260665349));
#62804=CARTESIAN_POINT('Ctrl Pts',(0.00828774270205792,-0.0307878597078928,
0.0723829167104463));
#62805=CARTESIAN_POINT('Ctrl Pts',(0.00782004690692066,-0.0308402475823424,
0.0723989617927675));
#62806=CARTESIAN_POINT('Ctrl Pts',(0.00701384657225643,-0.0309450233312383,
0.0727620400442508));
#62807=CARTESIAN_POINT('Ctrl Pts',(0.00668038516697007,-0.0309974112056886,
0.0731084553765258));
#62808=CARTESIAN_POINT('Ctrl Pts',(0.00635465831522934,-0.0311021869545879,
0.0739540130716083));
#62809=CARTESIAN_POINT('Ctrl Pts',(0.00636598244243914,-0.0311545748290377,
0.0744486796189194));
#62810=CARTESIAN_POINT('Ctrl Pts',(0.00671098369860905,-0.0312474112056882,
0.0751967969613253));
#62811=CARTESIAN_POINT('Ctrl Pts',(0.00696811726850124,-0.0312878597078925,
0.0754772937988554));
#62812=CARTESIAN_POINT('Ctrl Pts',(0.00760906327807618,-0.0313687567122965,
0.0758329541525405));
#62813=CARTESIAN_POINT('Ctrl Pts',(0.00799152536675427,-0.0314092052144999,
0.0759066312254608));
#62814=CARTESIAN_POINT('Ctrl Pts',(0.00873342443754237,-0.0314901022189058,
0.0758027496660232));
#62815=CARTESIAN_POINT('Ctrl Pts',(0.00909066570959304,-0.0315305507211086,
0.0756247584725279));
#62816=CARTESIAN_POINT('Ctrl Pts',(0.00962495708239995,-0.0316114477255139,
0.0750753379018474));
#62817=CARTESIAN_POINT('Ctrl Pts',(0.00979975975119023,-0.0316518962277159,
0.0747050174935392));
#62818=CARTESIAN_POINT('Ctrl Pts',(0.00986603384010217,-0.0317234272443419,
0.0740141973629227));
#62819=CARTESIAN_POINT('Ctrl Pts',(0.00981302274622929,-0.0317545097587632,
0.0737035212777265));
#62820=CARTESIAN_POINT('Ctrl Pts',(0.00968430513999177,-0.0317855922731845,
0.0734247205810942));
#62821=CARTESIAN_POINT('Ctrl Pts',(0.00814801668780212,-0.0203072579114564,
0.07605678506462));
#62822=CARTESIAN_POINT('Ctrl Pts',(0.00835212411518636,-0.0203255606965017,
0.076056125656151));
#62823=CARTESIAN_POINT('Ctrl Pts',(0.00855476749622787,-0.0203438634815471,
0.0760235656396361));
#62824=CARTESIAN_POINT('Ctrl Pts',(0.00939708426598712,-0.0204246662665928,
0.0757338805617789));
#62825=CARTESIAN_POINT('Ctrl Pts',(0.00988702802146066,-0.0204871662665918,
0.0751430794075642));
#62826=CARTESIAN_POINT('Ctrl Pts',(0.0101232087195095,-0.0206121662665931,
0.0738376922384734));
#62827=CARTESIAN_POINT('Ctrl Pts',(0.00987324480820894,-0.020674666266593,
0.073147689549446));
#62828=CARTESIAN_POINT('Ctrl Pts',(0.0089167610235679,-0.0207996662665919,
0.0722962388864693));
#62829=CARTESIAN_POINT('Ctrl Pts',(0.00822945225385138,-0.0208621662665925,
0.0721430341238275));
#62830=CARTESIAN_POINT('Ctrl Pts',(0.00703231984039108,-0.0209871662665924,
0.0724624609241718));
#62831=CARTESIAN_POINT('Ctrl Pts',(0.00653742293657822,-0.0210496662665924,
0.0729254531013723));
#62832=CARTESIAN_POINT('Ctrl Pts',(0.00612213906812888,-0.0211746662665925,
0.0740526572687589));
#62833=CARTESIAN_POINT('Ctrl Pts',(0.0062024986305861,-0.0212371662665924,
0.0747016337122979));
#62834=CARTESIAN_POINT('Ctrl Pts',(0.00683777690670826,-0.0213621662665925,
0.0756803008502788));
#62835=CARTESIAN_POINT('Ctrl Pts',(0.00738258273676963,-0.0214246662665922,
0.0760014915719832));
#62836=CARTESIAN_POINT('Ctrl Pts',(0.00851285299155973,-0.0215496662665927,
0.0761060218805955));
#62837=CARTESIAN_POINT('Ctrl Pts',(0.00908700825207452,-0.0216121662665926,
0.0758916126988471));
#62838=CARTESIAN_POINT('Ctrl Pts',(0.009867934505352,-0.0217371662665924,
0.0751086198167669));
#62839=CARTESIAN_POINT('Ctrl Pts',(0.0100698264375556,-0.0217996662665926,
0.0745489205445409));
#62840=CARTESIAN_POINT('Ctrl Pts',(0.00999137500636933,-0.0219246662665924,
0.0734730045098974));
#62841=CARTESIAN_POINT('Ctrl Pts',(0.00971409165292503,-0.0219871662665922,
0.0729652157409598));
#62842=CARTESIAN_POINT('Ctrl Pts',(0.00888282738880219,-0.0221121662665928,
0.0723178841967402));
#62843=CARTESIAN_POINT('Ctrl Pts',(0.00833621828939995,-0.022174666266592,
0.0721813898931065));
#62844=CARTESIAN_POINT('Ctrl Pts',(0.00731858981585824,-0.0222996662665929,
0.0723410721157334));
#62845=CARTESIAN_POINT('Ctrl Pts',(0.00685408613370773,-0.0223621662665927,
0.0726343422814147));
#62846=CARTESIAN_POINT('Ctrl Pts',(0.00627188449978499,-0.0224871662665922,
0.0734573086233949));
#62847=CARTESIAN_POINT('Ctrl Pts',(0.00615642736772064,-0.0225496662665926,
0.07398099780415));
#62848=CARTESIAN_POINT('Ctrl Pts',(0.00632058686144516,-0.0226746662665923,
0.0749546945714818));
#62849=CARTESIAN_POINT('Ctrl Pts',(0.00659784007307093,-0.0227371662665921,
0.0753994199917464));
#62850=CARTESIAN_POINT('Ctrl Pts',(0.007376147995406,-0.0228621662665928,
0.075974991173125));
#62851=CARTESIAN_POINT('Ctrl Pts',(0.00787234780121979,-0.0229246662665925,
0.0761038540413805));
#62852=CARTESIAN_POINT('Ctrl Pts',(0.00881571254739481,-0.0230496662665924,
0.0759944503948627));
#62853=CARTESIAN_POINT('Ctrl Pts',(0.00925841300542465,-0.0231121662665924,
0.0757578644326881));
#62854=CARTESIAN_POINT('Ctrl Pts',(0.0098711682512917,-0.0232371662665925,
0.0750551282138252));
#62855=CARTESIAN_POINT('Ctrl Pts',(0.0100392249004471,-0.0232996662665926,
0.0745928466798487));
#62856=CARTESIAN_POINT('Ctrl Pts',(0.0100319815915929,-0.0234246662665924,
0.0736769154324963));
#62857=CARTESIAN_POINT('Ctrl Pts',(0.0098576459212449,-0.0234871662665927,
0.0732271346566689));
#62858=CARTESIAN_POINT('Ctrl Pts',(0.00926368508465529,-0.0236121662665922,
0.0725504421633576));
#62859=CARTESIAN_POINT('Ctrl Pts',(0.00884704504328137,-0.0236746662665927,
0.0723256519701696));
#62860=CARTESIAN_POINT('Ctrl Pts',(0.00797138179410088,-0.0237996662665922,
0.07219343949548));
#62861=CARTESIAN_POINT('Ctrl Pts',(0.00751572112090685,-0.0238621662665923,
0.0722857508103344));
#62862=CARTESIAN_POINT('Ctrl Pts',(0.00676795485175628,-0.0239871662665926,
0.0727333505959289));
#62863=CARTESIAN_POINT('Ctrl Pts',(0.00647809666942974,-0.0240496662665925,
0.073086482268025));
#62864=CARTESIAN_POINT('Ctrl Pts',(0.00618146533527733,-0.0241746662665925,
0.0738916281021063));
#62865=CARTESIAN_POINT('Ctrl Pts',(0.00617506843092123,-0.0242371662665925,
0.0743407833313369));
#62866=CARTESIAN_POINT('Ctrl Pts',(0.00643703700353636,-0.0243621662665925,
0.0751443712971177));
#62867=CARTESIAN_POINT('Ctrl Pts',(0.00670404041284908,-0.0244246662665925,
0.0754965010570941));
#62868=CARTESIAN_POINT('Ctrl Pts',(0.00739271373153814,-0.0245496662665925,
0.0759650125972991));
#62869=CARTESIAN_POINT('Ctrl Pts',(0.00781207442037852,-0.0246121662665926,
0.0760804681250833));
#62870=CARTESIAN_POINT('Ctrl Pts',(0.00863215889728322,-0.0247371662665924,
0.0760382325197273));
#62871=CARTESIAN_POINT('Ctrl Pts',(0.0090306448835366,-0.024799666266592,
0.0758811474014697));
#62872=CARTESIAN_POINT('Ctrl Pts',(0.0096546204052879,-0.024924666266593,
0.0753648274104897));
#62873=CARTESIAN_POINT('Ctrl Pts',(0.00987876695480732,-0.0249871662665926,
0.0750072900452153));
#62874=CARTESIAN_POINT('Ctrl Pts',(0.0100752103419703,-0.0251121662665924,
0.0742327400711651));
#62875=CARTESIAN_POINT('Ctrl Pts',(0.0100474244538565,-0.0251746662665924,
0.0738177503330937));
#62876=CARTESIAN_POINT('Ctrl Pts',(0.00975897010215047,-0.0252996662665926,
0.0730837214741746));
#62877=CARTESIAN_POINT('Ctrl Pts',(0.00949934019014137,-0.0253621662665928,
0.0727662697552228));
#62878=CARTESIAN_POINT('Ctrl Pts',(0.00884867337874248,-0.0254871662665921,
0.0723385359604954));
#62879=CARTESIAN_POINT('Ctrl Pts',(0.00845929038676506,-0.0255496662665926,
0.0722289127955772));
#62880=CARTESIAN_POINT('Ctrl Pts',(0.00769050740141413,-0.0256746662665924,
0.0722485755987396));
#62881=CARTESIAN_POINT('Ctrl Pts',(0.0073127385103659,-0.0257371662665915,
0.0723774872479133));
#62882=CARTESIAN_POINT('Ctrl Pts',(0.00669672771899448,-0.0258621662665935,
0.0728221789114253));
#62883=CARTESIAN_POINT('Ctrl Pts',(0.00645955767124918,-0.0259246662665926,
0.0731368026319471));
#62884=CARTESIAN_POINT('Ctrl Pts',(0.00611222183958379,-0.0260919420154909,
0.0740795755859367));
#62885=CARTESIAN_POINT('Ctrl Pts',(0.00620960829772417,-0.0261967177643892,
0.0747851908841829));
#62886=CARTESIAN_POINT('Ctrl Pts',(0.00698099751955323,-0.0264062692621874,
0.0758117979253375));
#62887=CARTESIAN_POINT('Ctrl Pts',(0.00764579640796796,-0.0265110450110865,
0.0761138323326925));
#62888=CARTESIAN_POINT('Ctrl Pts',(0.00895151249954563,-0.0267205965088817,
0.0759939008582095));
#62889=CARTESIAN_POINT('Ctrl Pts',(0.00956921024717631,-0.0268253722577806,
0.0755695035082156));
#62890=CARTESIAN_POINT('Ctrl Pts',(0.0101391127975682,-0.0270349237555792,
0.0743566277259409));
#62891=CARTESIAN_POINT('Ctrl Pts',(0.0100758233948543,-0.0271396995044774,
0.0735890033938645));
#62892=CARTESIAN_POINT('Ctrl Pts',(0.00927465732816471,-0.0273492510022741,
0.0724764802177239));
#62893=CARTESIAN_POINT('Ctrl Pts',(0.00854863504798854,-0.0274540267511745,
0.0721581017954751));
#62894=CARTESIAN_POINT('Ctrl Pts',(0.0071586286123545,-0.0276635782489686,
0.0723565014738116));
#62895=CARTESIAN_POINT('Ctrl Pts',(0.00652722395860935,-0.0277683539978693,
0.0728754416319487));
#62896=CARTESIAN_POINT('Ctrl Pts',(0.0061941131930515,-0.0279255176212164,
0.0739025770922874));
#62897=CARTESIAN_POINT('Ctrl Pts',(0.00618172482778142,-0.0279779054956661,
0.0742791192866981));
#62898=CARTESIAN_POINT('Ctrl Pts',(0.00636558444125528,-0.0280826812445643,
0.0749848648164158));
#62899=CARTESIAN_POINT('Ctrl Pts',(0.00656179628659944,-0.0281350691190143,
0.0753127819778567));
#62900=CARTESIAN_POINT('Ctrl Pts',(0.0071076452778826,-0.028239844867912,
0.0758111224113399));
#62901=CARTESIAN_POINT('Ctrl Pts',(0.00745650463288417,-0.0282922327423619,
0.0759804115890255));
#62902=CARTESIAN_POINT('Ctrl Pts',(0.00819673799450679,-0.0283970084912602,
0.0760968804211664));
#62903=CARTESIAN_POINT('Ctrl Pts',(0.00858674947338286,-0.0284493963657099,
0.0760435018440831));
#62904=CARTESIAN_POINT('Ctrl Pts',(0.00927564963473071,-0.0285541721146081,
0.0757225423137761));
#62905=CARTESIAN_POINT('Ctrl Pts',(0.00957299018710003,-0.028606559989058,
0.0754552752219081));
#62906=CARTESIAN_POINT('Ctrl Pts',(0.00996560701721403,-0.0287113357379557,
0.0747915828297948));
#62907=CARTESIAN_POINT('Ctrl Pts',(0.010059696968687,-0.0287637236124047,
0.074396372440036));
#62908=CARTESIAN_POINT('Ctrl Pts',(0.0100007835149004,-0.0288684993613048,
0.0736158357642392));
#62909=CARTESIAN_POINT('Ctrl Pts',(0.00984747524688978,-0.0289208872357529,
0.073232313186738));
#62910=CARTESIAN_POINT('Ctrl Pts',(0.00933890234319653,-0.0290256629846524,
0.0726213568608565));
#62911=CARTESIAN_POINT('Ctrl Pts',(0.00898449292909369,-0.0290780508591023,
0.0723957035479018));
#62912=CARTESIAN_POINT('Ctrl Pts',(0.00820150519090858,-0.0291828266079989,
0.0721974790286785));
#62913=CARTESIAN_POINT('Ctrl Pts',(0.00777480494848981,-0.0292352144824501,
0.072225929314564));
#62914=CARTESIAN_POINT('Ctrl Pts',(0.00701567178618897,-0.0293399902313469,
0.0725388127232768));
#62915=CARTESIAN_POINT('Ctrl Pts',(0.00668553723143537,-0.029392378105796,
0.0728229295147053));
#62916=CARTESIAN_POINT('Ctrl Pts',(0.00626320349708927,-0.0294971538546968,
0.0735434428689412));
#62917=CARTESIAN_POINT('Ctrl Pts',(0.00617279507523841,-0.0295495417291453,
0.0739780598173242));
#62918=CARTESIAN_POINT('Ctrl Pts',(0.00628368831566111,-0.0296543174780434,
0.0748207970461326));
#62919=CARTESIAN_POINT('Ctrl Pts',(0.00648535233659179,-0.0297067053524937,
0.0752261858068767));
#62920=CARTESIAN_POINT('Ctrl Pts',(0.00710862553564354,-0.0298114811013907,
0.0758269273212183));
#62921=CARTESIAN_POINT('Ctrl Pts',(0.00752869276012381,-0.02986386897584,
0.0760196869779353));
#62922=CARTESIAN_POINT('Ctrl Pts',(0.00840797945427604,-0.0299686447247403,
0.076091415138353));
#62923=CARTESIAN_POINT('Ctrl Pts',(0.00886408949546226,-0.0300210325991884,
0.075969235922541));
#62924=CARTESIAN_POINT('Ctrl Pts',(0.00959764252618967,-0.0301258083480876,
0.0754482333981525));
#62925=CARTESIAN_POINT('Ctrl Pts',(0.00987164018299474,-0.0301781962225362,
0.0750506297150497));
#62926=CARTESIAN_POINT('Ctrl Pts',(0.0100900140080253,-0.0302829719714357,
0.07415859534242));
#62927=CARTESIAN_POINT('Ctrl Pts',(0.0100323696451357,-0.0303353598458849,
0.0736676702543576));
#62928=CARTESIAN_POINT('Ctrl Pts',(0.00959236173346572,-0.0304401355947827,
0.0728390376922328));
#62929=CARTESIAN_POINT('Ctrl Pts',(0.00921089015096985,-0.0304925234692313,
0.0725057397900231));
#62930=CARTESIAN_POINT('Ctrl Pts',(0.00830589411414326,-0.0305972992181321,
0.0721872899879916));
#62931=CARTESIAN_POINT('Ctrl Pts',(0.00778642158836204,-0.0306496870925817,
0.0722051113571944));
#62932=CARTESIAN_POINT('Ctrl Pts',(0.00689097003953919,-0.0307544628414776,
0.0726083845495457));
#62933=CARTESIAN_POINT('Ctrl Pts',(0.00652059245595663,-0.0308068507159279,
0.0729931501375565));
#62934=CARTESIAN_POINT('Ctrl Pts',(0.00615880568740368,-0.0309116264648272,
0.0739323161427358));
#62935=CARTESIAN_POINT('Ctrl Pts',(0.00617138346343902,-0.030964014339277,
0.0744817452447779));
#62936=CARTESIAN_POINT('Ctrl Pts',(0.00655457842863585,-0.0310568507159276,
0.0753126836656081));
#62937=CARTESIAN_POINT('Ctrl Pts',(0.00684017822748756,-0.0310972992181319,
0.0756242331860024));
#62938=CARTESIAN_POINT('Ctrl Pts',(0.00755208080592647,-0.0311781962225358,
0.0760192672747625));
#62939=CARTESIAN_POINT('Ctrl Pts',(0.0079768837425508,-0.0312186447247393,
0.0761011008417093));
#62940=CARTESIAN_POINT('Ctrl Pts',(0.00880091549178614,-0.0312995417291452,
0.0759857189703642));
#62941=CARTESIAN_POINT('Ctrl Pts',(0.00919770551606028,-0.031339990231348,
0.0757880230838218));
#62942=CARTESIAN_POINT('Ctrl Pts',(0.00979114614952519,-0.0314208872357532,
0.0751777783595053));
#62943=CARTESIAN_POINT('Ctrl Pts',(0.00998530052254685,-0.0314613357379553,
0.0747664612601165));
#62944=CARTESIAN_POINT('Ctrl Pts',(0.0100589115507385,-0.0315328667545812,
0.0739991631961976));
#62945=CARTESIAN_POINT('Ctrl Pts',(0.0100000318107133,-0.0315639492690025,
0.0736540934043486));
#62946=CARTESIAN_POINT('Ctrl Pts',(0.00985706439317406,-0.0315950317834238,
0.0733444277978263));
#62947=CARTESIAN_POINT('Ctrl Pts',(0.00815067148752137,-0.0203072579114564,
0.0762656663521488));
#62948=CARTESIAN_POINT('Ctrl Pts',(0.0083771381325318,-0.0203255606965017,
0.0762649347079084));
#62949=CARTESIAN_POINT('Ctrl Pts',(0.00860198035030984,-0.0203438634815471,
0.0762288078613937));
#62950=CARTESIAN_POINT('Ctrl Pts',(0.00953656982276594,-0.0204246662665928,
0.0759073888491967));
#62951=CARTESIAN_POINT('Ctrl Pts',(0.0100801851138304,-0.0204871662665918,
0.0752518676024789));
#62952=CARTESIAN_POINT('Ctrl Pts',(0.0103422385382883,-0.0206121662665931,
0.0738034800723812));
#62953=CARTESIAN_POINT('Ctrl Pts',(0.0100648920002843,-0.020674666266593,
0.0730378901277388));
#62954=CARTESIAN_POINT('Ctrl Pts',(0.00900362893656076,-0.0207996662665919,
0.0720931661776728));
#62955=CARTESIAN_POINT('Ctrl Pts',(0.008241028020177,-0.0208621662665925,
0.0719231783970233));
#62956=CARTESIAN_POINT('Ctrl Pts',(0.00691275415584957,-0.0209871662665924,
0.0722775972279668));
#62957=CARTESIAN_POINT('Ctrl Pts',(0.00636364311727103,-0.0210496662665924,
0.0727913084945308));
#62958=CARTESIAN_POINT('Ctrl Pts',(0.00590286642913209,-0.0211746662665925,
0.0740419937307385));
#62959=CARTESIAN_POINT('Ctrl Pts',(0.00599202908596152,-0.0212371662665924,
0.0747620631556615));
#62960=CARTESIAN_POINT('Ctrl Pts',(0.00669689975963152,-0.0213621662665925,
0.0758479396774564));
#62961=CARTESIAN_POINT('Ctrl Pts',(0.00730138706368173,-0.0214246662665922,
0.0762043156608544));
#62962=CARTESIAN_POINT('Ctrl Pts',(0.00855547426588603,-0.0215496662665927,
0.0763202968801402));
#62963=CARTESIAN_POINT('Ctrl Pts',(0.00919252612250013,-0.0216121662665926,
0.0760823999614819));
#62964=CARTESIAN_POINT('Ctrl Pts',(0.0100589999732895,-0.0217371662665924,
0.075213633090309));
#62965=CARTESIAN_POINT('Ctrl Pts',(0.0102830084237745,-0.0217996662665926,
0.0745926208223076));
#62966=CARTESIAN_POINT('Ctrl Pts',(0.0101959629269755,-0.0219246662665924,
0.0733988421450626));
#62967=CARTESIAN_POINT('Ctrl Pts',(0.00988830420246689,-0.0219871662665922,
0.0728354269849725));
#62968=CARTESIAN_POINT('Ctrl Pts',(0.00896597799697031,-0.0221121662665928,
0.0721171826520367));
#62969=CARTESIAN_POINT('Ctrl Pts',(0.00835948988205837,-0.022174666266592,
0.0719657358996911));
#62970=CARTESIAN_POINT('Ctrl Pts',(0.00723038395375605,-0.0222996662665929,
0.0721429107222321));
#62971=CARTESIAN_POINT('Ctrl Pts',(0.00671499560243656,-0.0223621662665927,
0.0724683075554325));
#62972=CARTESIAN_POINT('Ctrl Pts',(0.00606901592181546,-0.0224871662665922,
0.0733814268319492));
#62973=CARTESIAN_POINT('Ctrl Pts',(0.00594091088577522,-0.0225496662665926,
0.0739624842354635));
#62974=CARTESIAN_POINT('Ctrl Pts',(0.00612305344798784,-0.0226746662665923,
0.0750428459007938));
#62975=CARTESIAN_POINT('Ctrl Pts',(0.00643067872875265,-0.0227371662665921,
0.0755362893544149));
#62976=CARTESIAN_POINT('Ctrl Pts',(0.00729424742007936,-0.0228621662665928,
0.0761749122408133));
#62977=CARTESIAN_POINT('Ctrl Pts',(0.00784480408877878,-0.0229246662665925,
0.0763178915621161));
#62978=CARTESIAN_POINT('Ctrl Pts',(0.00889151097164585,-0.0230496662665924,
0.0761965031486893));
#62979=CARTESIAN_POINT('Ctrl Pts',(0.00938270763587042,-0.0231121662665924,
0.0759340000649118));
#62980=CARTESIAN_POINT('Ctrl Pts',(0.0100625879641978,-0.0232371662665925,
0.0751542816790953));
#62981=CARTESIAN_POINT('Ctrl Pts',(0.0102490546008787,-0.0232996662665926,
0.0746413589041057));
#62982=CARTESIAN_POINT('Ctrl Pts',(0.0102410178141923,-0.0234246662665924,
0.0736250907589115));
#62983=CARTESIAN_POINT('Ctrl Pts',(0.0100475843126518,-0.0234871662665927,
0.0731260381541277));
#62984=CARTESIAN_POINT('Ctrl Pts',(0.00938855725198137,-0.0236121662665922,
0.0723752164881653));
#62985=CARTESIAN_POINT('Ctrl Pts',(0.0089262758271642,-0.0236746662665927,
0.0721258013564626));
#62986=CARTESIAN_POINT('Ctrl Pts',(0.00795468689116961,-0.0237996662665922,
0.0719791054916663));
#62987=CARTESIAN_POINT('Ctrl Pts',(0.00744911026789867,-0.0238621662665923,
0.0720815291713897));
#62988=CARTESIAN_POINT('Ctrl Pts',(0.00661942895548025,-0.0239871662665926,
0.0725781618664859));
#62989=CARTESIAN_POINT('Ctrl Pts',(0.00629781787585632,-0.0240496662665925,
0.0729699778138594));
#62990=CARTESIAN_POINT('Ctrl Pts',(0.00596869167054677,-0.0241746662665925,
0.07386332441141));
#62991=CARTESIAN_POINT('Ctrl Pts',(0.00596159400885685,-0.0242371662665925,
0.0743616829432692));
#62992=CARTESIAN_POINT('Ctrl Pts',(0.00625226027464946,-0.0243621662665925,
0.0752533010137793));
#62993=CARTESIAN_POINT('Ctrl Pts',(0.0065485129249735,-0.0244246662665925,
0.0756440052932471));
#62994=CARTESIAN_POINT('Ctrl Pts',(0.00731262787164867,-0.0245496662665925,
0.0761638405487234));
#62995=CARTESIAN_POINT('Ctrl Pts',(0.00777792798085125,-0.0246121662665926,
0.0762919438047406));
#62996=CARTESIAN_POINT('Ctrl Pts',(0.00868784969457759,-0.0247371662665924,
0.07624508144423));
#62997=CARTESIAN_POINT('Ctrl Pts',(0.00912998835433636,-0.024799666266592,
0.0760707882292855));
#62998=CARTESIAN_POINT('Ctrl Pts',(0.00982231809848441,-0.024924666266593,
0.07549790728317));
#62999=CARTESIAN_POINT('Ctrl Pts',(0.010071019077723,-0.0249871662665926,
0.0751012030151419));
#63000=CARTESIAN_POINT('Ctrl Pts',(0.0102889821151069,-0.0251121662665924,
0.0742418039415068));
#63001=CARTESIAN_POINT('Ctrl Pts',(0.0102581523851926,-0.0251746662665924,
0.0737813536046464));
#63002=CARTESIAN_POINT('Ctrl Pts',(0.00993809892066803,-0.0252996662665926,
0.0729669145852015));
#63003=CARTESIAN_POINT('Ctrl Pts',(0.00965002750714532,-0.0253621662665928,
0.0726146871985494));
#63004=CARTESIAN_POINT('Ctrl Pts',(0.00892808254078336,-0.0254871662665921,
0.07214009674052));
#63005=CARTESIAN_POINT('Ctrl Pts',(0.00849604407482765,-0.0255496662665926,
0.0720184647612599));
#63006=CARTESIAN_POINT('Ctrl Pts',(0.00764304374228332,-0.0256746662665924,
0.0720402815521564));
#63007=CARTESIAN_POINT('Ctrl Pts',(0.00722389165927775,-0.0257371662665915,
0.0721833149981475));
#63008=CARTESIAN_POINT('Ctrl Pts',(0.00654039915241529,-0.0258621662665935,
0.0726767209970879));
#63009=CARTESIAN_POINT('Ctrl Pts',(0.00627724799864211,-0.0259246662665926,
0.0730258105884879));
#63010=CARTESIAN_POINT('Ctrl Pts',(0.00589186280469173,-0.0260919420154909,
0.0740718608505132));
#63011=CARTESIAN_POINT('Ctrl Pts',(0.00599991759097347,-0.0261967177643892,
0.0748547737082654));
#63012=CARTESIAN_POINT('Ctrl Pts',(0.00685580966361203,-0.0264062692621874,
0.0759938417732247));
#63013=CARTESIAN_POINT('Ctrl Pts',(0.00759343482402584,-0.0265110450110865,
0.0763289629385248));
#63014=CARTESIAN_POINT('Ctrl Pts',(0.00904218730885863,-0.0267205965088817,
0.0761958934123178));
#63015=CARTESIAN_POINT('Ctrl Pts',(0.00972755157183108,-0.0268253722577806,
0.0757250048942655));
#63016=CARTESIAN_POINT('Ctrl Pts',(0.010359884849577,-0.0270349237555792,
0.0743792630330001));
#63017=CARTESIAN_POINT('Ctrl Pts',(0.0102896623256786,-0.0271396995044774,
0.0735275482799331));
#63018=CARTESIAN_POINT('Ctrl Pts',(0.00940073146439328,-0.0273492510022741,
0.0722931522835415));
#63019=CARTESIAN_POINT('Ctrl Pts',(0.00859517611493118,-0.0274540267511745,
0.0719398966766563));
#63020=CARTESIAN_POINT('Ctrl Pts',(0.00705289958900958,-0.0276635782489686,
0.0721600303097132));
#63021=CARTESIAN_POINT('Ctrl Pts',(0.00635232687879448,-0.0277683539978693,
0.0727358184526565));
#63022=CARTESIAN_POINT('Ctrl Pts',(0.00598272505460037,-0.0279255176212164,
0.073875472823177));
#63023=CARTESIAN_POINT('Ctrl Pts',(0.00596897958949985,-0.0279779054956661,
0.0742932638294421));
#63024=CARTESIAN_POINT('Ctrl Pts',(0.00617298034709087,-0.0280826812445643,
0.0750763211850444));
#63025=CARTESIAN_POINT('Ctrl Pts',(0.00639068647810172,-0.0281350691190143,
0.075440160464901));
#63026=CARTESIAN_POINT('Ctrl Pts',(0.00699633121784709,-0.028239844867912,
0.0759930922591544));
#63027=CARTESIAN_POINT('Ctrl Pts',(0.00738340683150901,-0.0282922327423619,
0.0761809264433306));
#63028=CARTESIAN_POINT('Ctrl Pts',(0.00820473003409823,-0.0283970084912602,
0.076310154007468));
#63029=CARTESIAN_POINT('Ctrl Pts',(0.00863746583537968,-0.0284493963657099,
0.0762509280036797));
#63030=CARTESIAN_POINT('Ctrl Pts',(0.00940183247449225,-0.0285541721146081,
0.0758948085378461));
#63031=CARTESIAN_POINT('Ctrl Pts',(0.00973174559026465,-0.028606559989058,
0.0755982633195131));
#63032=CARTESIAN_POINT('Ctrl Pts',(0.0101673721494254,-0.0287113357379557,
0.0748618658679991));
#63033=CARTESIAN_POINT('Ctrl Pts',(0.0102717693088642,-0.0287637236124047,
0.0744233616342778));
#63034=CARTESIAN_POINT('Ctrl Pts',(0.0102064021029961,-0.0288684993613048,
0.0735573200377487));
#63035=CARTESIAN_POINT('Ctrl Pts',(0.0100362994783456,-0.0289208872357529,
0.0731317839731108));
#63036=CARTESIAN_POINT('Ctrl Pts',(0.00947201428442268,-0.0290256629846524,
0.072453899629834));
#63037=CARTESIAN_POINT('Ctrl Pts',(0.00907878062310723,-0.0290780508591023,
0.0722035268267701));
#63038=CARTESIAN_POINT('Ctrl Pts',(0.00821001945932422,-0.0291828266079989,
0.0719835875408627));
#63039=CARTESIAN_POINT('Ctrl Pts',(0.00773657577545569,-0.0292352144824501,
0.0720151544508798));
#63040=CARTESIAN_POINT('Ctrl Pts',(0.00689428236856863,-0.0293399902313469,
0.0723623130857159));
#63041=CARTESIAN_POINT('Ctrl Pts',(0.00652798278812114,-0.029392378105796,
0.0726775538261953));
#63042=CARTESIAN_POINT('Ctrl Pts',(0.00605938394721744,-0.0294971538546968,
0.0734769967671513));
#63043=CARTESIAN_POINT('Ctrl Pts',(0.00595907161542407,-0.0295495417291453,
0.0739592244029917));
#63044=CARTESIAN_POINT('Ctrl Pts',(0.00608211280228693,-0.0296543174780434,
0.0748942803942386));
#63045=CARTESIAN_POINT('Ctrl Pts',(0.00630586837465766,-0.0297067053524937,
0.0753440780020337));
#63046=CARTESIAN_POINT('Ctrl Pts',(0.00699741885923872,-0.0298114811013907,
0.0760106285387534));
#63047=CARTESIAN_POINT('Ctrl Pts',(0.00746350290246076,-0.02986386897584,
0.0762245043065757));
#63048=CARTESIAN_POINT('Ctrl Pts',(0.00843911221849071,-0.0299686447247403,
0.0763040900230327));
#63049=CARTESIAN_POINT('Ctrl Pts',(0.0089451874363639,-0.0300210325991884,
0.0761685265237053));
#63050=CARTESIAN_POINT('Ctrl Pts',(0.00975909850238958,-0.0301258083480876,
0.0755904500898765));
#63051=CARTESIAN_POINT('Ctrl Pts',(0.0100631115942824,-0.0301781962225362,
0.0751492903863319));
#63052=CARTESIAN_POINT('Ctrl Pts',(0.0103054074683059,-0.0302829719714357,
0.0741595369305542));
#63053=CARTESIAN_POINT('Ctrl Pts',(0.0102414483775728,-0.0303353598458849,
0.0736148328055268));
#63054=CARTESIAN_POINT('Ctrl Pts',(0.00975323921825422,-0.0304401355947827,
0.0726954265952984));
#63055=CARTESIAN_POINT('Ctrl Pts',(0.00932997882757754,-0.0304925234692313,
0.0723256171343211));
#63056=CARTESIAN_POINT('Ctrl Pts',(0.00832584380498464,-0.0305972992181321,
0.0719722823282605));
#63057=CARTESIAN_POINT('Ctrl Pts',(0.0077494649754808,-0.0306496870925817,
0.0719920559628832));
#63058=CARTESIAN_POINT('Ctrl Pts',(0.00675592000443203,-0.0307544628414776,
0.0724395062495526));
#63059=CARTESIAN_POINT('Ctrl Pts',(0.00634496891942769,-0.0308068507159279,
0.0728664214919276));
#63060=CARTESIAN_POINT('Ctrl Pts',(0.00594354974162806,-0.0309116264648272,
0.0739084696771727));
#63061=CARTESIAN_POINT('Ctrl Pts',(0.00595750536674637,-0.030964014339277,
0.0745180867156372));
#63062=CARTESIAN_POINT('Ctrl Pts',(0.00638267793035737,-0.0310568507159276,
0.0754400513829074));
#63063=CARTESIAN_POINT('Ctrl Pts',(0.00669956413626623,-0.0310972992181319,
0.0757857300068678));
#63064=CARTESIAN_POINT('Ctrl Pts',(0.00748945302262128,-0.0311781962225358,
0.0762240386264647));
#63065=CARTESIAN_POINT('Ctrl Pts',(0.00796079155782699,-0.0312186447247393,
0.0763148367595518));
#63066=CARTESIAN_POINT('Ctrl Pts',(0.00887509295304323,-0.0312995417291452,
0.0761868152287656));
#63067=CARTESIAN_POINT('Ctrl Pts',(0.00931534986442847,-0.031339990231348,
0.075967462485304));
#63068=CARTESIAN_POINT('Ctrl Pts',(0.00997379973563606,-0.0314208872357532,
0.0752903676969252));
#63069=CARTESIAN_POINT('Ctrl Pts',(0.0101892230058022,-0.0314613357379553,
0.0748339923228011));
#63070=CARTESIAN_POINT('Ctrl Pts',(0.0102708978512695,-0.0315328667545812,
0.0739826395793677));
#63071=CARTESIAN_POINT('Ctrl Pts',(0.0102055680523813,-0.0315639492690025,
0.0735997686615574));
#63072=CARTESIAN_POINT('Ctrl Pts',(0.0100469390803206,-0.0315950317834238,
0.0732561803273014));
#63073=CARTESIAN_POINT('',(0.0102415292846688,-0.0315281082229192,0.0740373581220502));
#63074=CARTESIAN_POINT('Ctrl Pts',(0.0102415292846687,-0.0315281082229192,
0.0740373581220493));
#63075=CARTESIAN_POINT('Ctrl Pts',(0.0102443061585269,-0.0315281082229192,
0.0740372104215577));
#63076=CARTESIAN_POINT('Ctrl Pts',(0.0102470791223289,-0.0315281082229192,
0.0740374674812331));
#63077=CARTESIAN_POINT('Ctrl Pts',(0.0102549222898814,-0.0315281082229192,
0.0740392868388633));
#63078=CARTESIAN_POINT('Ctrl Pts',(0.0102596737838761,-0.0315281082229192,
0.0740416912990496));
#63079=CARTESIAN_POINT('Ctrl Pts',(0.0102714431960483,-0.0315281082229192,
0.0740498637422819));
#63080=CARTESIAN_POINT('Ctrl Pts',(0.0102781083576007,-0.0315281082229192,
0.0740571642570058));
#63081=CARTESIAN_POINT('Ctrl Pts',(0.01029611995105,-0.0315281082229192,
0.0740808578266151));
#63082=CARTESIAN_POINT('Ctrl Pts',(0.0103082953978233,-0.0315281082229192,
0.0741042852756716));
#63083=CARTESIAN_POINT('Ctrl Pts',(0.0103375938004529,-0.0315281082229192,
0.0741803459859531));
#63084=CARTESIAN_POINT('Ctrl Pts',(0.0103535661419107,-0.0315281082229192,
0.0742431662099169));
#63085=CARTESIAN_POINT('Ctrl Pts',(0.0103867339291107,-0.0315281082229192,
0.0744813090868569));
#63086=CARTESIAN_POINT('Ctrl Pts',(0.0103828904157489,-0.0315281082229192,
0.074698144384189));
#63087=CARTESIAN_POINT('Ctrl Pts',(0.0102634625434987,-0.0315281082229192,
0.075190809856021));
#63088=CARTESIAN_POINT('Ctrl Pts',(0.0101565404905841,-0.0315281082229192,
0.0754290476681851));
#63089=CARTESIAN_POINT('Ctrl Pts',(0.0098125654375786,-0.0315281082229192,
0.0759373966430771));
#63090=CARTESIAN_POINT('Ctrl Pts',(0.00958025235175371,-0.0315281082229192,
0.0761276005840903));
#63091=CARTESIAN_POINT('Ctrl Pts',(0.00916609298882152,-0.0315281082229192,
0.0764086558067814));
#63092=CARTESIAN_POINT('Ctrl Pts',(0.00889372820965532,-0.0315281082229192,
0.0765284368321801));
#63093=CARTESIAN_POINT('Ctrl Pts',(0.00822455503474282,-0.0315281082229192,
0.0766836549896214));
#63094=CARTESIAN_POINT('Ctrl Pts',(0.00789635708856245,-0.0315281082229192,
0.0766587650478001));
#63095=CARTESIAN_POINT('Ctrl Pts',(0.00745899885480862,-0.0315281082229192,
0.0765870776260973));
#63096=CARTESIAN_POINT('Ctrl Pts',(0.0071495560914034,-0.0315281082229192,
0.0765064246987785));
#63097=CARTESIAN_POINT('Ctrl Pts',(0.00655000913918567,-0.0315281082229192,
0.0761454330379778));
#63098=CARTESIAN_POINT('Ctrl Pts',(0.00630893772584743,-0.0315281082317243,
0.0759248089475972));
#63099=CARTESIAN_POINT('Ctrl Pts',(0.00611837819382198,-0.0315281082317243,
0.0756651070488126));
#63100=CARTESIAN_POINT('Ctrl Pts',(0.00599688119407085,-0.0315281082317243,
0.0754995262395158));
#63101=CARTESIAN_POINT('Ctrl Pts',(0.00584236692428051,-0.0315281082229192,
0.0752474041328658));
#63102=CARTESIAN_POINT('Ctrl Pts',(0.00567647591673654,-0.0315281082229192,
0.0746524710000351));
#63103=CARTESIAN_POINT('Ctrl Pts',(0.00564801698991816,-0.0315281082229192,
0.0743893561988201));
#63104=CARTESIAN_POINT('Ctrl Pts',(0.00567898251827618,-0.0315281082229192,
0.0738464149833142));
#63105=CARTESIAN_POINT('Ctrl Pts',(0.00574582072759108,-0.0315281082229192,
0.0735505592342265));
#63106=CARTESIAN_POINT('Ctrl Pts',(0.00600663983621015,-0.0315281082229192,
0.0730144137359113));
#63107=CARTESIAN_POINT('Ctrl Pts',(0.00617508989093895,-0.0315281082229192,
0.0727998376780962));
#63108=CARTESIAN_POINT('Ctrl Pts',(0.00651170243980347,-0.0315281082229192,
0.07250050147065));
#63109=CARTESIAN_POINT('Ctrl Pts',(0.00666205465774635,-0.0315281082229192,
0.0724117683127483));
#63110=CARTESIAN_POINT('Ctrl Pts',(0.00683725022531139,-0.0315281082229192,
0.0723411242055322));
#63111=CARTESIAN_POINT('Ctrl Pts',(0.00688753578065855,-0.0315281082229192,
0.0723272897287553));
#63112=CARTESIAN_POINT('Ctrl Pts',(0.00694306395763103,-0.0315281082229192,
0.0723209583585516));
#63113=CARTESIAN_POINT('Ctrl Pts',(0.00696094236000387,-0.0315281082229192,
0.0723202174840268));
#63114=CARTESIAN_POINT('Ctrl Pts',(0.0069840622333989,-0.0315281082229192,
0.0723240830795569));
#63115=CARTESIAN_POINT('Ctrl Pts',(0.00699153257991565,-0.0315281082229192,
0.072326114864887));
#63116=CARTESIAN_POINT('Ctrl Pts',(0.00700236736391432,-0.0315281082229192,
0.0723317082934015));
#63117=CARTESIAN_POINT('Ctrl Pts',(0.00700628093475598,-0.0315281082229192,
0.0723344806504444));
#63118=CARTESIAN_POINT('Ctrl Pts',(0.00701259234411832,-0.0315281082229192,
0.0723413281190414));
#63119=CARTESIAN_POINT('Ctrl Pts',(0.00701488997279872,-0.0315281082229192,
0.0723451142719038));
#63120=CARTESIAN_POINT('Ctrl Pts',(0.00701838111679472,-0.0315281082229192,
0.0723547226865156));
#63121=CARTESIAN_POINT('Ctrl Pts',(0.00701901723954043,-0.0315281082229192,
0.0723604498449024));
#63122=CARTESIAN_POINT('Ctrl Pts',(0.00701855552816112,-0.0315281082229192,
0.0723749667362874));
#63123=CARTESIAN_POINT('Ctrl Pts',(0.00701633056667769,-0.0315281082229192,
0.0723844150799716));
#63124=CARTESIAN_POINT('Ctrl Pts',(0.00700533444282857,-0.0315281082229192,
0.07241623739993));
#63125=CARTESIAN_POINT('Ctrl Pts',(0.006990685757266,-0.0315281082229192,
0.0724418345314411));
#63126=CARTESIAN_POINT('Ctrl Pts',(0.00689688702227869,-0.0315281082229192,
0.0725877915328833));
#63127=CARTESIAN_POINT('Ctrl Pts',(0.00673080378851581,-0.0315281082229192,
0.0727773871144422));
#63128=CARTESIAN_POINT('Ctrl Pts',(0.00645755406311322,-0.0315281082229192,
0.0732998343171583));
#63129=CARTESIAN_POINT('Ctrl Pts',(0.00639422129915112,-0.0315281082229192,
0.0735231500021576));
#63130=CARTESIAN_POINT('Ctrl Pts',(0.00632988803870339,-0.0315281082229192,
0.0739546853543993));
#63131=CARTESIAN_POINT('Ctrl Pts',(0.00633656673913058,-0.0315281082229192,
0.0741967633645283));
#63132=CARTESIAN_POINT('Ctrl Pts',(0.00643779274399072,-0.0315281082229192,
0.0746675424839583));
#63133=CARTESIAN_POINT('Ctrl Pts',(0.00652881158812033,-0.0315281082229192,
0.0748790244316244));
#63134=CARTESIAN_POINT('Ctrl Pts',(0.00678360157726101,-0.0315281082229192,
0.0752602394191017));
#63135=CARTESIAN_POINT('Ctrl Pts',(0.00694815581386843,-0.0315281082229192,
0.0754289690043338));
#63136=CARTESIAN_POINT('Ctrl Pts',(0.00737024253118045,-0.0315281082229192,
0.0757225788008902));
#63137=CARTESIAN_POINT('Ctrl Pts',(0.00760228849775194,-0.0315281082229192,
0.0758044262461883));
#63138=CARTESIAN_POINT('Ctrl Pts',(0.00799226788849764,-0.0315281082229192,
0.0758882741543255));
#63139=CARTESIAN_POINT('Ctrl Pts',(0.00824055843794205,-0.0315281082229192,
0.0759101885441291));
#63140=CARTESIAN_POINT('Ctrl Pts',(0.00877222168832291,-0.0315281082229192,
0.0758096151203664));
#63141=CARTESIAN_POINT('Ctrl Pts',(0.00901072440531448,-0.031528108222919,
0.0757123703062191));
#63142=CARTESIAN_POINT('Ctrl Pts',(0.00942936166701739,-0.031528108222919,
0.0754370419824175));
#63143=CARTESIAN_POINT('Ctrl Pts',(0.00961497183389103,-0.0315281082229192,
0.075259295977966));
#63144=CARTESIAN_POINT('Ctrl Pts',(0.00998728974756363,-0.0315281082229192,
0.0747160970557801));
#63145=CARTESIAN_POINT('Ctrl Pts',(0.0100770415748213,-0.0315281082229192,
0.0744130626439684));
#63146=CARTESIAN_POINT('Ctrl Pts',(0.0101559062218069,-0.0315281082229192,
0.0741709433951502));
#63147=CARTESIAN_POINT('Ctrl Pts',(0.0101731338183302,-0.0315281082229192,
0.0741211717490925));
#63148=CARTESIAN_POINT('Ctrl Pts',(0.0101976354678072,-0.0315281082229192,
0.0740742120961429));
#63149=CARTESIAN_POINT('Ctrl Pts',(0.010205012267356,-0.0315281082229192,
0.0740623410869319));
#63150=CARTESIAN_POINT('Ctrl Pts',(0.0102172281970335,-0.0315281082229192,
0.0740489929183199));
#63151=CARTESIAN_POINT('Ctrl Pts',(0.0102218571970461,-0.0315281082229192,
0.0740448431008829));
#63152=CARTESIAN_POINT('Ctrl Pts',(0.0102305223709339,-0.0315281082229192,
0.0740398720236682));
#63153=CARTESIAN_POINT('Ctrl Pts',(0.0102342438738187,-0.0315281082229192,
0.0740384012812181));
#63154=CARTESIAN_POINT('Ctrl Pts',(0.0102393236553668,-0.0315281082229192,
0.0740375392238714));
#63155=CARTESIAN_POINT('Ctrl Pts',(0.0102404267778191,-0.0315281082229192,
0.0740374167638213));
#63156=CARTESIAN_POINT('Ctrl Pts',(0.0102415292846687,-0.0315281082229192,
0.0740373581220493));
#63157=CARTESIAN_POINT('',(0.00600748819723868,-0.0211741814719622,0.0740583944593496));
#63158=CARTESIAN_POINT('Ctrl Pts',(0.0102415292846701,-0.0315281082229191,
0.0740373581220501));
#63159=CARTESIAN_POINT('Ctrl Pts',(0.0102474107028906,-0.0315193335619991,
0.0741426793323997));
#63160=CARTESIAN_POINT('Ctrl Pts',(0.0102454265162678,-0.0315105589010791,
0.0742481447151113));
#63161=CARTESIAN_POINT('Ctrl Pts',(0.0101892230058022,-0.0314613357379553,
0.0748339923228011));
#63162=CARTESIAN_POINT('Ctrl Pts',(0.00997379973563606,-0.0314208872357532,
0.0752903676969252));
#63163=CARTESIAN_POINT('Ctrl Pts',(0.00931534986442847,-0.031339990231348,
0.075967462485304));
#63164=CARTESIAN_POINT('Ctrl Pts',(0.00887509295304323,-0.0312995417291452,
0.0761868152287656));
#63165=CARTESIAN_POINT('Ctrl Pts',(0.00796079155782699,-0.0312186447247393,
0.0763148367595518));
#63166=CARTESIAN_POINT('Ctrl Pts',(0.00748945302262128,-0.0311781962225358,
0.0762240386264647));
#63167=CARTESIAN_POINT('Ctrl Pts',(0.00669956413626623,-0.0310972992181319,
0.0757857300068678));
#63168=CARTESIAN_POINT('Ctrl Pts',(0.00638267793035737,-0.0310568507159276,
0.0754400513829074));
#63169=CARTESIAN_POINT('Ctrl Pts',(0.00595750536674637,-0.030964014339277,
0.0745180867156372));
#63170=CARTESIAN_POINT('Ctrl Pts',(0.00594354974162806,-0.0309116264648272,
0.0739084696771727));
#63171=CARTESIAN_POINT('Ctrl Pts',(0.00634496891942769,-0.0308068507159279,
0.0728664214919276));
#63172=CARTESIAN_POINT('Ctrl Pts',(0.00675592000443203,-0.0307544628414776,
0.0724395062495526));
#63173=CARTESIAN_POINT('Ctrl Pts',(0.0077494649754808,-0.0306496870925817,
0.0719920559628832));
#63174=CARTESIAN_POINT('Ctrl Pts',(0.00832584380498464,-0.0305972992181321,
0.0719722823282605));
#63175=CARTESIAN_POINT('Ctrl Pts',(0.00932997882757754,-0.0304925234692313,
0.0723256171343211));
#63176=CARTESIAN_POINT('Ctrl Pts',(0.00975323921825422,-0.0304401355947827,
0.0726954265952984));
#63177=CARTESIAN_POINT('Ctrl Pts',(0.0102414483775728,-0.0303353598458849,
0.0736148328055268));
#63178=CARTESIAN_POINT('Ctrl Pts',(0.0103054074683059,-0.0302829719714357,
0.0741595369305542));
#63179=CARTESIAN_POINT('Ctrl Pts',(0.0100631115942824,-0.0301781962225362,
0.0751492903863319));
#63180=CARTESIAN_POINT('Ctrl Pts',(0.00975909850238958,-0.0301258083480876,
0.0755904500898765));
#63181=CARTESIAN_POINT('Ctrl Pts',(0.0089451874363639,-0.0300210325991884,
0.0761685265237053));
#63182=CARTESIAN_POINT('Ctrl Pts',(0.00843911221849071,-0.0299686447247403,
0.0763040900230327));
#63183=CARTESIAN_POINT('Ctrl Pts',(0.00746350290246076,-0.02986386897584,
0.0762245043065757));
#63184=CARTESIAN_POINT('Ctrl Pts',(0.00699741885923872,-0.0298114811013907,
0.0760106285387534));
#63185=CARTESIAN_POINT('Ctrl Pts',(0.00630586837465766,-0.0297067053524937,
0.0753440780020337));
#63186=CARTESIAN_POINT('Ctrl Pts',(0.00608211280228693,-0.0296543174780434,
0.0748942803942386));
#63187=CARTESIAN_POINT('Ctrl Pts',(0.00595907161542407,-0.0295495417291453,
0.0739592244029917));
#63188=CARTESIAN_POINT('Ctrl Pts',(0.00605938394721744,-0.0294971538546968,
0.0734769967671513));
#63189=CARTESIAN_POINT('Ctrl Pts',(0.00652798278812114,-0.029392378105796,
0.0726775538261953));
#63190=CARTESIAN_POINT('Ctrl Pts',(0.00689428236856863,-0.0293399902313469,
0.0723623130857159));
#63191=CARTESIAN_POINT('Ctrl Pts',(0.00773657577545569,-0.0292352144824501,
0.0720151544508798));
#63192=CARTESIAN_POINT('Ctrl Pts',(0.00821001945932422,-0.0291828266079989,
0.0719835875408627));
#63193=CARTESIAN_POINT('Ctrl Pts',(0.00907878062310723,-0.0290780508591023,
0.0722035268267701));
#63194=CARTESIAN_POINT('Ctrl Pts',(0.00947201428442268,-0.0290256629846524,
0.072453899629834));
#63195=CARTESIAN_POINT('Ctrl Pts',(0.0100362994783456,-0.0289208872357529,
0.0731317839731108));
#63196=CARTESIAN_POINT('Ctrl Pts',(0.0102064021029961,-0.0288684993613048,
0.0735573200377487));
#63197=CARTESIAN_POINT('Ctrl Pts',(0.0102717693088642,-0.0287637236124047,
0.0744233616342778));
#63198=CARTESIAN_POINT('Ctrl Pts',(0.0101673721494254,-0.0287113357379557,
0.0748618658679991));
#63199=CARTESIAN_POINT('Ctrl Pts',(0.00973174559026465,-0.028606559989058,
0.0755982633195131));
#63200=CARTESIAN_POINT('Ctrl Pts',(0.00940183247449225,-0.0285541721146081,
0.0758948085378461));
#63201=CARTESIAN_POINT('Ctrl Pts',(0.00863746583537968,-0.0284493963657099,
0.0762509280036797));
#63202=CARTESIAN_POINT('Ctrl Pts',(0.00820473003409823,-0.0283970084912602,
0.076310154007468));
#63203=CARTESIAN_POINT('Ctrl Pts',(0.00738340683150901,-0.0282922327423619,
0.0761809264433306));
#63204=CARTESIAN_POINT('Ctrl Pts',(0.00699633121784709,-0.028239844867912,
0.0759930922591544));
#63205=CARTESIAN_POINT('Ctrl Pts',(0.00639068647810172,-0.0281350691190143,
0.075440160464901));
#63206=CARTESIAN_POINT('Ctrl Pts',(0.00617298034709087,-0.0280826812445643,
0.0750763211850444));
#63207=CARTESIAN_POINT('Ctrl Pts',(0.00596897958949985,-0.0279779054956661,
0.0742932638294421));
#63208=CARTESIAN_POINT('Ctrl Pts',(0.00598272505460037,-0.0279255176212164,
0.073875472823177));
#63209=CARTESIAN_POINT('Ctrl Pts',(0.00635232687879448,-0.0277683539978693,
0.0727358184526565));
#63210=CARTESIAN_POINT('Ctrl Pts',(0.00705289958900958,-0.0276635782489686,
0.0721600303097132));
#63211=CARTESIAN_POINT('Ctrl Pts',(0.00859517611493118,-0.0274540267511745,
0.0719398966766563));
#63212=CARTESIAN_POINT('Ctrl Pts',(0.00940073146439328,-0.0273492510022741,
0.0722931522835415));
#63213=CARTESIAN_POINT('Ctrl Pts',(0.0102896623256786,-0.0271396995044774,
0.0735275482799331));
#63214=CARTESIAN_POINT('Ctrl Pts',(0.010359884849577,-0.0270349237555792,
0.0743792630330001));
#63215=CARTESIAN_POINT('Ctrl Pts',(0.00972755157183108,-0.0268253722577806,
0.0757250048942655));
#63216=CARTESIAN_POINT('Ctrl Pts',(0.00904218730885863,-0.0267205965088817,
0.0761958934123178));
#63217=CARTESIAN_POINT('Ctrl Pts',(0.00759343482402584,-0.0265110450110865,
0.0763289629385248));
#63218=CARTESIAN_POINT('Ctrl Pts',(0.00685580966361203,-0.0264062692621874,
0.0759938417732247));
#63219=CARTESIAN_POINT('Ctrl Pts',(0.00599991759097347,-0.0261967177643892,
0.0748547737082654));
#63220=CARTESIAN_POINT('Ctrl Pts',(0.00589186280469173,-0.0260919420154909,
0.0740718608505132));
#63221=CARTESIAN_POINT('Ctrl Pts',(0.00627724799864211,-0.0259246662665926,
0.0730258105884879));
#63222=CARTESIAN_POINT('Ctrl Pts',(0.00654039915241529,-0.0258621662665935,
0.0726767209970879));
#63223=CARTESIAN_POINT('Ctrl Pts',(0.00722389165927775,-0.0257371662665915,
0.0721833149981475));
#63224=CARTESIAN_POINT('Ctrl Pts',(0.00764304374228332,-0.0256746662665924,
0.0720402815521564));
#63225=CARTESIAN_POINT('Ctrl Pts',(0.00849604407482765,-0.0255496662665926,
0.0720184647612599));
#63226=CARTESIAN_POINT('Ctrl Pts',(0.00892808254078336,-0.0254871662665921,
0.07214009674052));
#63227=CARTESIAN_POINT('Ctrl Pts',(0.00965002750714532,-0.0253621662665928,
0.0726146871985494));
#63228=CARTESIAN_POINT('Ctrl Pts',(0.00993809892066803,-0.0252996662665926,
0.0729669145852015));
#63229=CARTESIAN_POINT('Ctrl Pts',(0.0102581523851926,-0.0251746662665924,
0.0737813536046464));
#63230=CARTESIAN_POINT('Ctrl Pts',(0.0102889821151069,-0.0251121662665924,
0.0742418039415068));
#63231=CARTESIAN_POINT('Ctrl Pts',(0.010071019077723,-0.0249871662665926,
0.0751012030151419));
#63232=CARTESIAN_POINT('Ctrl Pts',(0.00982231809848441,-0.024924666266593,
0.07549790728317));
#63233=CARTESIAN_POINT('Ctrl Pts',(0.00912998835433636,-0.024799666266592,
0.0760707882292855));
#63234=CARTESIAN_POINT('Ctrl Pts',(0.00868784969457759,-0.0247371662665924,
0.07624508144423));
#63235=CARTESIAN_POINT('Ctrl Pts',(0.00777792798085125,-0.0246121662665926,
0.0762919438047406));
#63236=CARTESIAN_POINT('Ctrl Pts',(0.00731262787164867,-0.0245496662665925,
0.0761638405487234));
#63237=CARTESIAN_POINT('Ctrl Pts',(0.0065485129249735,-0.0244246662665925,
0.0756440052932471));
#63238=CARTESIAN_POINT('Ctrl Pts',(0.00625226027464946,-0.0243621662665925,
0.0752533010137793));
#63239=CARTESIAN_POINT('Ctrl Pts',(0.00596159400885685,-0.0242371662665925,
0.0743616829432692));
#63240=CARTESIAN_POINT('Ctrl Pts',(0.00596869167054677,-0.0241746662665925,
0.07386332441141));
#63241=CARTESIAN_POINT('Ctrl Pts',(0.00629781787585632,-0.0240496662665925,
0.0729699778138594));
#63242=CARTESIAN_POINT('Ctrl Pts',(0.00661942895548025,-0.0239871662665926,
0.0725781618664859));
#63243=CARTESIAN_POINT('Ctrl Pts',(0.00744911026789867,-0.0238621662665923,
0.0720815291713897));
#63244=CARTESIAN_POINT('Ctrl Pts',(0.00795468689116961,-0.0237996662665922,
0.0719791054916663));
#63245=CARTESIAN_POINT('Ctrl Pts',(0.0089262758271642,-0.0236746662665927,
0.0721258013564626));
#63246=CARTESIAN_POINT('Ctrl Pts',(0.00938855725198137,-0.0236121662665922,
0.0723752164881653));
#63247=CARTESIAN_POINT('Ctrl Pts',(0.0100475843126518,-0.0234871662665927,
0.0731260381541277));
#63248=CARTESIAN_POINT('Ctrl Pts',(0.0102410178141923,-0.0234246662665924,
0.0736250907589115));
#63249=CARTESIAN_POINT('Ctrl Pts',(0.0102490546008787,-0.0232996662665926,
0.0746413589041057));
#63250=CARTESIAN_POINT('Ctrl Pts',(0.0100625879641978,-0.0232371662665925,
0.0751542816790953));
#63251=CARTESIAN_POINT('Ctrl Pts',(0.00938270763587042,-0.0231121662665924,
0.0759340000649118));
#63252=CARTESIAN_POINT('Ctrl Pts',(0.00889151097164585,-0.0230496662665924,
0.0761965031486893));
#63253=CARTESIAN_POINT('Ctrl Pts',(0.00784480408877878,-0.0229246662665925,
0.0763178915621161));
#63254=CARTESIAN_POINT('Ctrl Pts',(0.00729424742007936,-0.0228621662665928,
0.0761749122408133));
#63255=CARTESIAN_POINT('Ctrl Pts',(0.00643067872875265,-0.0227371662665921,
0.0755362893544149));
#63256=CARTESIAN_POINT('Ctrl Pts',(0.00612305344798784,-0.0226746662665923,
0.0750428459007938));
#63257=CARTESIAN_POINT('Ctrl Pts',(0.00594091088577522,-0.0225496662665926,
0.0739624842354635));
#63258=CARTESIAN_POINT('Ctrl Pts',(0.00606901592181546,-0.0224871662665922,
0.0733814268319492));
#63259=CARTESIAN_POINT('Ctrl Pts',(0.00671499560243656,-0.0223621662665927,
0.0724683075554325));
#63260=CARTESIAN_POINT('Ctrl Pts',(0.00723038395375605,-0.0222996662665929,
0.0721429107222321));
#63261=CARTESIAN_POINT('Ctrl Pts',(0.00835948988205837,-0.022174666266592,
0.0719657358996911));
#63262=CARTESIAN_POINT('Ctrl Pts',(0.00896597799697031,-0.0221121662665928,
0.0721171826520367));
#63263=CARTESIAN_POINT('Ctrl Pts',(0.00988830420246689,-0.0219871662665922,
0.0728354269849725));
#63264=CARTESIAN_POINT('Ctrl Pts',(0.0101959629269755,-0.0219246662665924,
0.0733988421450626));
#63265=CARTESIAN_POINT('Ctrl Pts',(0.0102830084237745,-0.0217996662665926,
0.0745926208223076));
#63266=CARTESIAN_POINT('Ctrl Pts',(0.0100589999732895,-0.0217371662665924,
0.075213633090309));
#63267=CARTESIAN_POINT('Ctrl Pts',(0.00919252612250013,-0.0216121662665926,
0.0760823999614819));
#63268=CARTESIAN_POINT('Ctrl Pts',(0.00855547426588603,-0.0215496662665927,
0.0763202968801402));
#63269=CARTESIAN_POINT('Ctrl Pts',(0.00730138706368173,-0.0214246662665922,
0.0762043156608544));
#63270=CARTESIAN_POINT('Ctrl Pts',(0.00669689975963152,-0.0213621662665925,
0.0758479396774564));
#63271=CARTESIAN_POINT('Ctrl Pts',(0.00610859628485939,-0.0212578380017156,
0.0749416387703421));
#63272=CARTESIAN_POINT('Ctrl Pts',(0.00599064760068548,-0.0212160097368389,
0.0744989393311625));
#63273=CARTESIAN_POINT('Ctrl Pts',(0.00600748819723773,-0.0211741814719621,
0.0740583944593496));
#63274=CARTESIAN_POINT('',(0.00895037744954432,-0.0211741814719619,0.0761032845693596));
#63275=CARTESIAN_POINT('Ctrl Pts',(0.00895037744954477,-0.0211741814719619,
0.0761032845693594));
#63276=CARTESIAN_POINT('Ctrl Pts',(0.00895142341614423,-0.0211741814719619,
0.0761057562390223));
#63277=CARTESIAN_POINT('Ctrl Pts',(0.00895279546040267,-0.0211741814719619,
0.0761080260384607));
#63278=CARTESIAN_POINT('Ctrl Pts',(0.0089562501401301,-0.0211741814719619,
0.0761123590771521));
#63279=CARTESIAN_POINT('Ctrl Pts',(0.00895832322888189,-0.0211741814719619,
0.0761143334593383));
#63280=CARTESIAN_POINT('Ctrl Pts',(0.00896593439949515,-0.0211741814719619,
0.0761202179010537));
#63281=CARTESIAN_POINT('Ctrl Pts',(0.00897242564316084,-0.0211741814719619,
0.076123153785668));
#63282=CARTESIAN_POINT('Ctrl Pts',(0.00899823396132728,-0.0211741814719619,
0.0761316568472288));
#63283=CARTESIAN_POINT('Ctrl Pts',(0.00902247926375369,-0.0211741814719619,
0.0761323854854028));
#63284=CARTESIAN_POINT('Ctrl Pts',(0.00909067528635312,-0.0211741814719619,
0.0761310837812301));
#63285=CARTESIAN_POINT('Ctrl Pts',(0.00916256604711786,-0.0211741814719619,
0.0761179828307763));
#63286=CARTESIAN_POINT('Ctrl Pts',(0.0094044630434647,-0.0211741814719619,
0.0760382388246817));
#63287=CARTESIAN_POINT('Ctrl Pts',(0.00960115375427539,-0.0211741814719619,
0.0759369373400467));
#63288=CARTESIAN_POINT('Ctrl Pts',(0.00999901075226726,-0.0211741814719619,
0.0756042971860892));
#63289=CARTESIAN_POINT('Ctrl Pts',(0.010168666941163,-0.0211741814719619,
0.0753988227592878));
#63290=CARTESIAN_POINT('Ctrl Pts',(0.0104152222765945,-0.0211741814719619,
0.0749673473278423));
#63291=CARTESIAN_POINT('Ctrl Pts',(0.0105190162621075,-0.0211741814719619,
0.0747132809438133));
#63292=CARTESIAN_POINT('Ctrl Pts',(0.0106108249011952,-0.0211741814719619,
0.0741008079828946));
#63293=CARTESIAN_POINT('Ctrl Pts',(0.0105931415034016,-0.0211741814719619,
0.0737885844705757));
#63294=CARTESIAN_POINT('Ctrl Pts',(0.0104463470744042,-0.0211741814719619,
0.0731922680894886));
#63295=CARTESIAN_POINT('Ctrl Pts',(0.0103180576222123,-0.0211741814719619,
0.0729082566766417));
#63296=CARTESIAN_POINT('Ctrl Pts',(0.0099644329500286,-0.0211741814719619,
0.0724044777589146));
#63297=CARTESIAN_POINT('Ctrl Pts',(0.00974294206368656,-0.0211741814719619,
0.0721926834393527));
#63298=CARTESIAN_POINT('Ctrl Pts',(0.00920576807857105,-0.0211741814719619,
0.0718531426457546));
#63299=CARTESIAN_POINT('Ctrl Pts',(0.00889561756514791,-0.0211741814719619,
0.071736241382821));
#63300=CARTESIAN_POINT('Ctrl Pts',(0.00827174092211097,-0.0211741814719619,
0.071630329583783));
#63301=CARTESIAN_POINT('Ctrl Pts',(0.00795886823722732,-0.0211741814719619,
0.0716346314104874));
#63302=CARTESIAN_POINT('Ctrl Pts',(0.00734095337665573,-0.0211741814719619,
0.0717688073312937));
#63303=CARTESIAN_POINT('Ctrl Pts',(0.00708575460295718,-0.0211741814719619,
0.071895244930667));
#63304=CARTESIAN_POINT('Ctrl Pts',(0.006653901489938,-0.0211741814719619,
0.072179942485354));
#63305=CARTESIAN_POINT('Ctrl Pts',(0.00644724510751011,-0.0211741814719619,
0.0723766081242654));
#63306=CARTESIAN_POINT('Ctrl Pts',(0.00612446840762261,-0.0211741814719619,
0.0728227795090391));
#63307=CARTESIAN_POINT('Ctrl Pts',(0.0060148726041794,-0.0211741814719619,
0.0730573587817859));
#63308=CARTESIAN_POINT('Ctrl Pts',(0.00589812726791177,-0.0211741814719619,
0.0735089027067287));
#63309=CARTESIAN_POINT('Ctrl Pts',(0.00589346761698436,-0.0211741814719619,
0.0736999278899219));
#63310=CARTESIAN_POINT('Ctrl Pts',(0.00591824566295887,-0.0211741814719619,
0.0739041184431284));
#63311=CARTESIAN_POINT('Ctrl Pts',(0.00593298868605388,-0.0211741814719619,
0.0739614758718291));
#63312=CARTESIAN_POINT('Ctrl Pts',(0.005957576476281,-0.0211741814719619,
0.0740152647149347));
#63313=CARTESIAN_POINT('Ctrl Pts',(0.00596672380209973,-0.0211741814719619,
0.0740316468526178));
#63314=CARTESIAN_POINT('Ctrl Pts',(0.0059823803419084,-0.0211741814719619,
0.0740475599562614));
#63315=CARTESIAN_POINT('Ctrl Pts',(0.00598722794163848,-0.0211741814719619,
0.0740514990739912));
#63316=CARTESIAN_POINT('Ctrl Pts',(0.00599498500208107,-0.0211741814719619,
0.0740554998710154));
#63317=CARTESIAN_POINT('Ctrl Pts',(0.00599745107590697,-0.0211741814719619,
0.0740564951510525));
#63318=CARTESIAN_POINT('Ctrl Pts',(0.00600246497103547,-0.0211741814719619,
0.0740578817256914));
#63319=CARTESIAN_POINT('Ctrl Pts',(0.00600494927171444,-0.0211741814719619,
0.0740582845598504));
#63320=CARTESIAN_POINT('Ctrl Pts',(0.00600748819723879,-0.0211741814719619,
0.0740583944593472));
#63321=CARTESIAN_POINT('Ctrl Pts',(0.00600748819723879,-0.0211741814719619,
0.0740583944593471));
#63322=CARTESIAN_POINT('Ctrl Pts',(0.00601070231456546,-0.0211741814719619,
0.074058533585081));
#63323=CARTESIAN_POINT('Ctrl Pts',(0.00601386573624221,-0.0211741814719619,
0.0740581967876821));
#63324=CARTESIAN_POINT('Ctrl Pts',(0.00602032959859923,-0.0211741814719619,
0.0740566385094979));
#63325=CARTESIAN_POINT('Ctrl Pts',(0.00602353437818118,-0.0211741814719619,
0.0740553792170983));
#63326=CARTESIAN_POINT('Ctrl Pts',(0.00603379822221034,-0.0211741814719619,
0.074050110918832));
#63327=CARTESIAN_POINT('Ctrl Pts',(0.00604038521610018,-0.0211741814719619,
0.0740445702503871));
#63328=CARTESIAN_POINT('Ctrl Pts',(0.00605963783788561,-0.0211741814719619,
0.0740249955212598));
#63329=CARTESIAN_POINT('Ctrl Pts',(0.00607311807020041,-0.0211741814719619,
0.0740046692333217));
#63330=CARTESIAN_POINT('Ctrl Pts',(0.0061160806526335,-0.0211741814719619,
0.0739272008086412));
#63331=CARTESIAN_POINT('Ctrl Pts',(0.00614780156907989,-0.0211741814719619,
0.0738518940925071));
#63332=CARTESIAN_POINT('Ctrl Pts',(0.00626308582369267,-0.0211741814719619,
0.073595816618586));
#63333=CARTESIAN_POINT('Ctrl Pts',(0.00636873577430343,-0.0211741814719619,
0.0733776720079871));
#63334=CARTESIAN_POINT('Ctrl Pts',(0.00670988430688753,-0.0211741814719619,
0.0729655110110068));
#63335=CARTESIAN_POINT('Ctrl Pts',(0.00689489702552421,-0.0211741814719619,
0.0728047622729589));
#63336=CARTESIAN_POINT('Ctrl Pts',(0.00729018071586256,-0.0211741814719619,
0.0725694044020097));
#63337=CARTESIAN_POINT('Ctrl Pts',(0.00749475094614348,-0.0211741814719619,
0.0724887144709966));
#63338=CARTESIAN_POINT('Ctrl Pts',(0.00794565217078984,-0.0211741814719619,
0.072401913681025));
#63339=CARTESIAN_POINT('Ctrl Pts',(0.00819205162095311,-0.0211741814719622,
0.0724054295806454));
#63340=CARTESIAN_POINT('Ctrl Pts',(0.0086533508659248,-0.0211741814719622,
0.0724992888967247));
#63341=CARTESIAN_POINT('Ctrl Pts',(0.0088699157664898,-0.0211741814719563,
0.072585266090591));
#63342=CARTESIAN_POINT('Ctrl Pts',(0.00924694454333932,-0.0211741814719563,
0.0728259648510416));
#63343=CARTESIAN_POINT('Ctrl Pts',(0.00941528697237473,-0.0211741814719619,
0.0729802370505302));
#63344=CARTESIAN_POINT('Ctrl Pts',(0.00969406333781521,-0.0211741814719619,
0.0733800321346033));
#63345=CARTESIAN_POINT('Ctrl Pts',(0.00979247324332182,-0.0211741814719619,
0.0736000915629057));
#63346=CARTESIAN_POINT('Ctrl Pts',(0.00988871785872756,-0.0211741814719619,
0.0739957305323329));
#63347=CARTESIAN_POINT('Ctrl Pts',(0.00992783454669963,-0.0211741814719619,
0.0742476174138145));
#63348=CARTESIAN_POINT('Ctrl Pts',(0.00984789973010626,-0.0211741814719619,
0.0747689103030387));
#63349=CARTESIAN_POINT('Ctrl Pts',(0.00977449732126798,-0.0211741814719619,
0.074980541548417));
#63350=CARTESIAN_POINT('Ctrl Pts',(0.00953289899259933,-0.0211741814719619,
0.0754403783588731));
#63351=CARTESIAN_POINT('Ctrl Pts',(0.00936282454286502,-0.0211741814719619,
0.0756352637677106));
#63352=CARTESIAN_POINT('Ctrl Pts',(0.00914639631262419,-0.0211741814719619,
0.075858559708378));
#63353=CARTESIAN_POINT('Ctrl Pts',(0.00906928299020927,-0.0211741814719619,
0.0759289651434673));
#63354=CARTESIAN_POINT('Ctrl Pts',(0.00899184880715194,-0.0211741814719619,
0.0760111053919389));
#63355=CARTESIAN_POINT('Ctrl Pts',(0.00897214521593804,-0.0211741814719619,
0.0760346209492319));
#63356=CARTESIAN_POINT('Ctrl Pts',(0.00895510134701174,-0.0211741814719619,
0.0760638173989724));
#63357=CARTESIAN_POINT('Ctrl Pts',(0.00895089982051269,-0.0211741814719619,
0.0760730008099204));
#63358=CARTESIAN_POINT('Ctrl Pts',(0.0089482497709946,-0.0211741814719619,
0.0760855423549168));
#63359=CARTESIAN_POINT('Ctrl Pts',(0.00894784735747076,-0.0211741814719619,
0.0760894012590408));
#63360=CARTESIAN_POINT('Ctrl Pts',(0.00894829061504419,-0.0211741814719619,
0.0760967100289629));
#63361=CARTESIAN_POINT('Ctrl Pts',(0.00894901845018085,-0.0211741814719619,
0.0761000731881343));
#63362=CARTESIAN_POINT('Ctrl Pts',(0.00895037744954474,-0.0211741814719619,
0.0761032845693594));
#63363=CARTESIAN_POINT('Origin',(-0.0248134380203094,-0.0211741814719619,
0.00872990597260584));
#63364=CARTESIAN_POINT('Origin',(0.000869198225586133,-0.0315281082229192,
0.0821343473622993));
#107889=UNCERTAINTY_MEASURE_WITH_UNIT(LENGTH_MEASURE(1.E-5),#107911,
'DISTANCE_ACCURACY_VALUE',
'Maximum model space distance between geometric entities at asserted c
onnectivities');
#107898=UNCERTAINTY_MEASURE_WITH_UNIT(LENGTH_MEASURE(1.E-5),#107911,
'DISTANCE_ACCURACY_VALUE',
'Maximum model space distance between geometric entities at asserted c
onnectivities');
#107901=(
GEOMETRIC_REPRESENTATION_CONTEXT(3)
GLOBAL_UNCERTAINTY_ASSIGNED_CONTEXT((#107889))
GLOBAL_UNIT_ASSIGNED_CONTEXT((#107911,#107912,#107913))
REPRESENTATION_CONTEXT('','3D')
);
#107910=(
GEOMETRIC_REPRESENTATION_CONTEXT(3)
GLOBAL_UNCERTAINTY_ASSIGNED_CONTEXT((#107898))
GLOBAL_UNIT_ASSIGNED_CONTEXT((#107911,#107912,#107913))
REPRESENTATION_CONTEXT('','3D')
);
#107911=(
LENGTH_UNIT()
NAMED_UNIT(*)
SI_UNIT($,.METRE.)
);
#107912=(
NAMED_UNIT(*)
PLANE_ANGLE_UNIT()
SI_UNIT($,.RADIAN.)
);
#107913=(
NAMED_UNIT(*)
SI_UNIT($,.STERADIAN.)
SOLID_ANGLE_UNIT()
);
#107916=SHAPE_DEFINITION_REPRESENTATION(#107927,#107948);
#107927=PRODUCT_DEFINITION_SHAPE('',$,#107960);
#107948=SHAPE_REPRESENTATION('',(#45668),#107901);
#107957=PRODUCT_DEFINITION_CONTEXT('part definition',#107992,'design');
#107960=PRODUCT_DEFINITION('Tension Spring','Tension Spring',#107971,#107957);
#107971=PRODUCT_DEFINITION_FORMATION('',$,#107996);
#107992=APPLICATION_CONTEXT('Managed model based 3d engineering');
#107993=PRODUCT_CONTEXT('part definition',#107992,'mechanical');
#107996=PRODUCT('Tension Spring','Tension Spring',
'LEGAL AND USAGE DISCLAIMER: this Data/Model is provided \X2\201C\X0\A
S IS\X2\201D\X0\ for informational and representational only. It is a 
geometric approximation and is NOT engineered, certified, or guarantee
d for dimensional accuracy, exact tolerances, or production-level prec
ision. Vendor disclaims all implied warranties including fitness for a
 particular purpose. DO NOT USE FOR DIRECT PHYSICAL MANUFACTURING, AUT
OMATED PRODUCTION, OR SAFETY-CRITICAL SYSTEMS without independent engi
neering verification and resolution of any design discrepancies.',(#107993));
#108007=PRESENTATION_STYLE_ASSIGNMENT((#108014));
#108014=SURFACE_STYLE_USAGE(.BOTH.,#108021);
#108021=SURFACE_SIDE_STYLE('',(#108028));
#108028=SURFACE_STYLE_FILL_AREA(#108035);
#108035=FILL_AREA_STYLE('Opaque(48,59,150)',(#108042));
#108042=FILL_AREA_STYLE_COLOUR('Opaque(48,59,150)',#108049);
#108049=COLOUR_RGB('Opaque(48,59,150)',0.188235294117647,0.231372549019608,
0.588235294117647);
ENDSEC;
END-ISO-10303-21;
